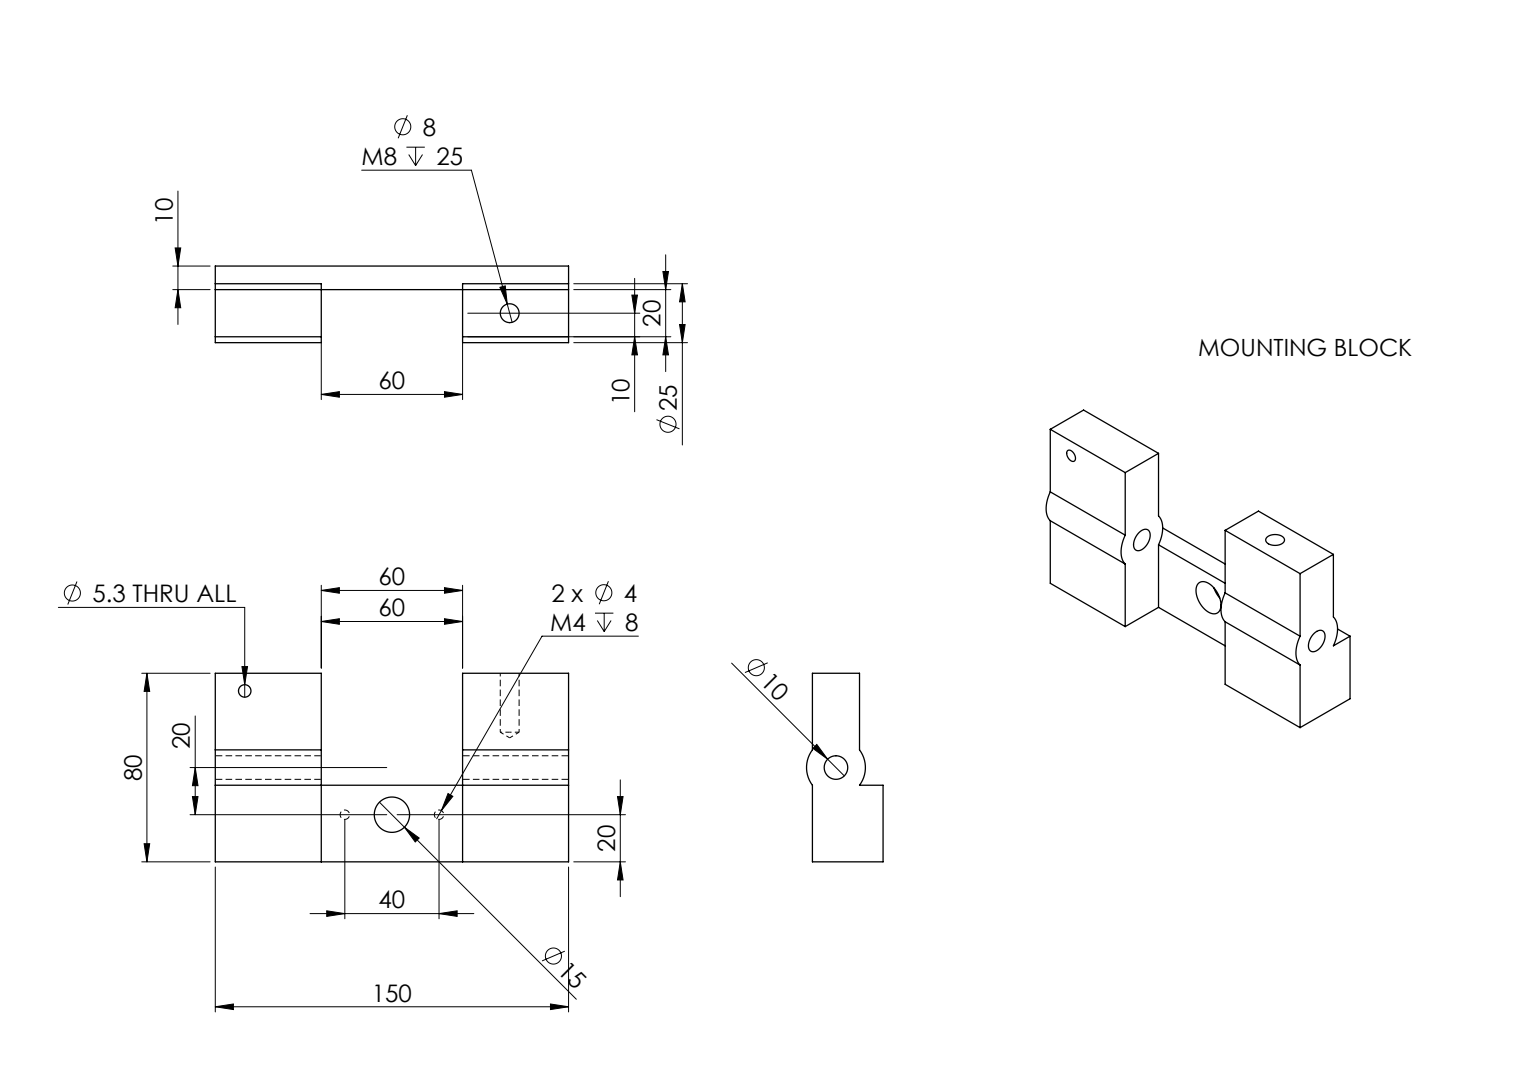
ISO-10303-21;
HEADER;
FILE_DESCRIPTION (('STEP AP214'),
    '1' );
FILE_NAME ('Mounting block.step',
    '2026-10-25T07:12:54',
    ( '' ),
    ( '' ),
    'SwSTEP 2.0',
    'SolidWorks 2026',
    '' );
FILE_SCHEMA (( 'AUTOMOTIVE_DESIGN' ));
ENDSEC;

DATA;
#10=ORIENTED_EDGE ( 'NONE', *, *, #6895, .T. ) ;
#23=DIRECTION ( 'NONE',  ( 1.000000000000000000, 3.469446951953615668E-16, -0.000000000000000000 ) ) ;
#24=DIRECTION ( 'NONE',  ( -1.000000000000000000, 9.251858538542972814E-17, -0.000000000000000000 ) ) ;
#32=FACE_OUTER_BOUND ( 'NONE', #8639, .T. ) ;
#35=VECTOR ( 'NONE', #3248, 1000.000000000000000 ) ;
#47=VECTOR ( 'NONE', #619, 1000.000000000000000 ) ;
#67=EDGE_LOOP ( 'NONE', ( #6510, #1768, #3467, #950 ) ) ;
#82=PLANE ( 'NONE',  #5621 ) ;
#101=ORIENTED_EDGE ( 'NONE', *, *, #5437, .F. ) ;
#111=LINE ( 'NONE', #5314, #1494 ) ;
#116=EDGE_LOOP ( 'NONE', ( #1810, #12426, #10336 ) ) ;
#132=EDGE_CURVE ( 'NONE', #594, #13026, #10926, .T. ) ;
#134=EDGE_CURVE ( 'NONE', #822, #8082, #1591, .T. ) ;
#137=CARTESIAN_POINT ( 'NONE',  ( 50.00000000000000000, 40.00000000000000000, 0.000000000000000000 ) ) ;
#141=CARTESIAN_POINT ( 'NONE',  ( -75.00000000000001421, -5.000000000000025757, 6.123233995736775157E-16 ) ) ;
#152=FACE_OUTER_BOUND ( 'NONE', #7758, .T. ) ;
#163=ADVANCED_FACE ( 'NONE', ( #12857 ), #1236, .F. ) ;
#167=CARTESIAN_POINT ( 'NONE',  ( -75.00000000000001421, -2.602085213965211904E-14, 0.000000000000000000 ) ) ;
#183=FACE_OUTER_BOUND ( 'NONE', #3328, .T. ) ;
#207=VECTOR ( 'NONE', #526, 1000.000000000000000 ) ;
#211=ORIENTED_EDGE ( 'NONE', *, *, #8650, .F. ) ;
#216=EDGE_CURVE ( 'NONE', #11745, #13576, #7487, .T. ) ;
#218=CIRCLE ( 'NONE', #6639, 5.000000000000000000 ) ;
#236=FACE_OUTER_BOUND ( 'NONE', #5614, .T. ) ;
#241=CARTESIAN_POINT ( 'NONE',  ( -30.00000000000000000, 7.499999999999991118, 10.00000000000000000 ) ) ;
#246=VECTOR ( 'NONE', #11169, 1000.000000000000000 ) ;
#251=CARTESIAN_POINT ( 'NONE',  ( 20.00000000000000000, -20.00000000000000000, -12.00000000000000000 ) ) ;
#255=CARTESIAN_POINT ( 'NONE',  ( 75.00000000000001421, 2.602085213965211904E-14, 0.000000000000000000 ) ) ;
#264=ADVANCED_FACE ( 'NONE', ( #3266 ), #5618, .F. ) ;
#293=ORIENTED_EDGE ( 'NONE', *, *, #1456, .F. ) ;
#298=DIRECTION ( 'NONE',  ( 1.000000000000000000, 0.000000000000000000, 0.000000000000000000 ) ) ;
#312=AXIS2_PLACEMENT_3D ( 'NONE', #6238, #11325, #3101 ) ;
#314=DIRECTION ( 'NONE',  ( -0.000000000000000000, -0.000000000000000000, -1.000000000000000000 ) ) ;
#361=ORIENTED_EDGE ( 'NONE', *, *, #4832, .F. ) ;
#366=CARTESIAN_POINT ( 'NONE',  ( -75.00000000000001421, -2.602085213965211904E-14, 0.000000000000000000 ) ) ;
#376=ORIENTED_EDGE ( 'NONE', *, *, #3505, .F. ) ;
#377=ORIENTED_EDGE ( 'NONE', *, *, #754, .F. ) ;
#391=DIRECTION ( 'NONE',  ( 1.000000000000000000, 3.469446951953615175E-16, 0.000000000000000000 ) ) ;
#404=AXIS2_PLACEMENT_3D ( 'NONE', #167, #4383, #2039 ) ;
#419=ORIENTED_EDGE ( 'NONE', *, *, #10834, .F. ) ;
#423=ORIENTED_EDGE ( 'NONE', *, *, #11853, .T. ) ;
#427=EDGE_CURVE ( 'NONE', #5687, #966, #2944, .T. ) ;
#430=AXIS2_PLACEMENT_3D ( 'NONE', #5828, #10990, #3471 ) ;
#440=APPLICATION_CONTEXT ( 'automotive_design' ) ;
#447=CARTESIAN_POINT ( 'NONE',  ( -62.49999999999997158, 32.50000000000001421, 15.00000000000000000 ) ) ;
#448=FACE_OUTER_BOUND ( 'NONE', #5406, .T. ) ;
#450=CARTESIAN_POINT ( 'NONE',  ( 0.000000000000000000, 0.000000000000000000, -10.00000000000000000 ) ) ;
#457=ORIENTED_EDGE ( 'NONE', *, *, #5953, .F. ) ;
#497=EDGE_CURVE ( 'NONE', #9340, #10627, #13638, .T. ) ;
#515=CARTESIAN_POINT ( 'NONE',  ( 30.00000000000000355, -40.00000000000000000, 10.00000000000000000 ) ) ;
#526=DIRECTION ( 'NONE',  ( -0.000000000000000000, -0.000000000000000000, -1.000000000000000000 ) ) ;
#551=FACE_OUTER_BOUND ( 'NONE', #4902, .T. ) ;
#581=CARTESIAN_POINT ( 'NONE',  ( 50.00000000000000000, 40.00000000000000000, 4.000000000000003553 ) ) ;
#583=CARTESIAN_POINT ( 'NONE',  ( -30.00000000000000000, -39.99999999999998579, -10.00000000000000000 ) ) ;
#594=VERTEX_POINT ( 'NONE', #8606 ) ;
#597=CIRCLE ( 'NONE', #11881, 12.50000000000000000 ) ;
#619=DIRECTION ( 'NONE',  ( -0.000000000000000000, -0.000000000000000000, 1.000000000000000000 ) ) ;
#640=DIRECTION ( 'NONE',  ( 1.000000000000000000, 0.000000000000000000, 0.000000000000000000 ) ) ;
#668=EDGE_CURVE ( 'NONE', #3281, #8692, #12777, .T. ) ;
#669=ORIENTED_EDGE ( 'NONE', *, *, #12070, .F. ) ;
#686=VERTEX_POINT ( 'NONE', #2504 ) ;
#699=CARTESIAN_POINT ( 'NONE',  ( 30.00000000000000355, -40.00000000000000000, 0.000000000000000000 ) ) ;
#715=DIRECTION ( 'NONE',  ( -1.000000000000000000, 0.000000000000000000, -0.000000000000000000 ) ) ;
#720=VERTEX_POINT ( 'NONE', #9842 ) ;
#723=ORIENTED_EDGE ( 'NONE', *, *, #9205, .T. ) ;
#726=CIRCLE ( 'NONE', #7603, 2.649999999999985700 ) ;
#738=ORIENTED_EDGE ( 'NONE', *, *, #10743, .T. ) ;
#754=EDGE_CURVE ( 'NONE', #9622, #4847, #5703, .T. ) ;
#771=CARTESIAN_POINT ( 'NONE',  ( 2.449293598294706513E-15, -20.00000000000000000, -20.00000000000000000 ) ) ;
#822=VERTEX_POINT ( 'NONE', #5907 ) ;
#830=AXIS2_PLACEMENT_3D ( 'NONE', #11462, #2962, #13381 ) ;
#859=CARTESIAN_POINT ( 'NONE',  ( 30.00000000000000355, 0.000000000000000000, -10.00000000000000000 ) ) ;
#871=FACE_OUTER_BOUND ( 'NONE', #4942, .T. ) ;
#877=AXIS2_PLACEMENT_3D ( 'NONE', #137, #12911, #3388 ) ;
#885=AXIS2_PLACEMENT_3D ( 'NONE', #1429, #5608, #5539 ) ;
#897=ORIENTED_EDGE ( 'NONE', *, *, #668, .F. ) ;
#931=ADVANCED_FACE ( 'NONE', ( #12055 ), #11004, .F. ) ;
#936=ADVANCED_FACE ( 'NONE', ( #551 ), #3748, .F. ) ;
#939=VECTOR ( 'NONE', #6527, 999.9999999999998863 ) ;
#941=EDGE_LOOP ( 'NONE', ( #8309, #9440 ) ) ;
#944=DIRECTION ( 'NONE',  ( -0.000000000000000000, -0.000000000000000000, -1.000000000000000000 ) ) ;
#950=ORIENTED_EDGE ( 'NONE', *, *, #3505, .T. ) ;
#953=LINE ( 'NONE', #9544, #6686 ) ;
#966=VERTEX_POINT ( 'NONE', #3845 ) ;
#985=ORIENTED_EDGE ( 'NONE', *, *, #7880, .F. ) ;
#991=CARTESIAN_POINT ( 'NONE',  ( -22.00000000000000000, -19.99999999999999289, -20.00000000000000000 ) ) ;
#1004=DIRECTION ( 'NONE',  ( -0.000000000000000000, 1.000000000000000000, -0.000000000000000000 ) ) ;
#1009=VECTOR ( 'NONE', #6135, 1000.000000000000114 ) ;
#1051=DIRECTION ( 'NONE',  ( -1.000000000000000000, 0.000000000000000000, 0.000000000000000000 ) ) ;
#1071=DIRECTION ( 'NONE',  ( 0.000000000000000000, 1.000000000000000000, 0.000000000000000000 ) ) ;
#1091=EDGE_CURVE ( 'NONE', #5946, #5030, #9628, .T. ) ;
#1120=FACE_BOUND ( 'NONE', #6057, .T. ) ;
#1134=FACE_BOUND ( 'NONE', #8492, .T. ) ;
#1135=EDGE_CURVE ( 'NONE', #11879, #2319, #10522, .T. ) ;
#1140=ORIENTED_EDGE ( 'NONE', *, *, #3820, .F. ) ;
#1156=VECTOR ( 'NONE', #12886, 1000.000000000000000 ) ;
#1158=EDGE_CURVE ( 'NONE', #8508, #7078, #7834, .T. ) ;
#1167=LINE ( 'NONE', #8721, #8679 ) ;
#1186=ORIENTED_EDGE ( 'NONE', *, *, #10636, .T. ) ;
#1188=DIRECTION ( 'NONE',  ( -3.469446951953614682E-16, 1.000000000000000000, 0.000000000000000000 ) ) ;
#1196=EDGE_CURVE ( 'NONE', #4847, #8976, #4787, .T. ) ;
#1214=CARTESIAN_POINT ( 'NONE',  ( 0.000000000000000000, 0.000000000000000000, -10.00000000000000000 ) ) ;
#1218=DIRECTION ( 'NONE',  ( 1.000000000000000000, 3.469446951953615175E-16, 0.000000000000000000 ) ) ;
#1226=EDGE_CURVE ( 'NONE', #11270, #10506, #4928, .T. ) ;
#1227=PLANE ( 'NONE',  #1317 ) ;
#1232=ORIENTED_EDGE ( 'NONE', *, *, #1226, .T. ) ;
#1236=CYLINDRICAL_SURFACE ( 'NONE', #7578, 4.000000000000003553 ) ;
#1257=ADVANCED_FACE ( 'NONE', ( #12380 ), #8937, .T. ) ;
#1274=CARTESIAN_POINT ( 'NONE',  ( 30.00000000000000355, -40.00000000000000000, 10.00000000000000000 ) ) ;
#1288=AXIS2_PLACEMENT_3D ( 'NONE', #11344, #5061, #6175 ) ;
#1290=VECTOR ( 'NONE', #1188, 1000.000000000000000 ) ;
#1291=FACE_BOUND ( 'NONE', #2165, .T. ) ;
#1317=AXIS2_PLACEMENT_3D ( 'NONE', #5473, #1427, #6575 ) ;
#1328=EDGE_CURVE ( 'NONE', #11270, #8976, #8325, .T. ) ;
#1340=CARTESIAN_POINT ( 'NONE',  ( 7.500000000000003553, -20.00000000000000000, -10.00000000000000000 ) ) ;
#1349=CARTESIAN_POINT ( 'NONE',  ( -20.00000000000000000, -19.99999999999999289, -12.00000000000000000 ) ) ;
#1375=( NAMED_UNIT ( * ) PLANE_ANGLE_UNIT ( ) SI_UNIT ( $, .RADIAN. ) );
#1382=DIRECTION ( 'NONE',  ( -0.000000000000000000, -0.000000000000000000, 1.000000000000000000 ) ) ;
#1384=VERTEX_POINT ( 'NONE', #10512 ) ;
#1394=AXIS2_PLACEMENT_3D ( 'NONE', #5354, #11635, #6333 ) ;
#1400=ORIENTED_EDGE ( 'NONE', *, *, #11817, .F. ) ;
#1413=CARTESIAN_POINT ( 'NONE',  ( -18.00000000000000355, -19.99999999999999289, -12.00000000000000000 ) ) ;
#1426=EDGE_CURVE ( 'NONE', #11691, #3041, #5274, .T. ) ;
#1427=DIRECTION ( 'NONE',  ( 1.000000000000000000, -0.000000000000000000, 0.000000000000000000 ) ) ;
#1429=CARTESIAN_POINT ( 'NONE',  ( -20.00000000000000000, -19.99999999999999289, -20.00000000000000000 ) ) ;
#1436=EDGE_LOOP ( 'NONE', ( #11212, #8239, #723, #12909 ) ) ;
#1442=DIRECTION ( 'NONE',  ( 0.000000000000000000, -1.000000000000000000, -0.000000000000000000 ) ) ;
#1444=SURFACE_SIDE_STYLE ('',( #12107 ) ) ;
#1452=DIRECTION ( 'NONE',  ( 1.000000000000000000, 3.469446951953615175E-16, 0.000000000000000000 ) ) ;
#1456=EDGE_CURVE ( 'NONE', #11270, #13379, #3187, .T. ) ;
#1461=DIRECTION ( 'NONE',  ( 1.000000000000000000, 3.469446951953615668E-16, -0.000000000000000000 ) ) ;
#1478=FACE_OUTER_BOUND ( 'NONE', #9905, .T. ) ;
#1484=VECTOR ( 'NONE', #9958, 1000.000000000000000 ) ;
#1486=ORIENTED_EDGE ( 'NONE', *, *, #1877, .F. ) ;
#1488=DIRECTION ( 'NONE',  ( 0.8571673013836855759, 1.049727191973305147E-16, -0.5150380737757258576 ) ) ;
#1494=VECTOR ( 'NONE', #3161, 1000.000000000000000 ) ;
#1496=LINE ( 'NONE', #9945, #8636 ) ;
#1523=FACE_OUTER_BOUND ( 'NONE', #4743, .T. ) ;
#1534=MECHANICAL_DESIGN_GEOMETRIC_PRESENTATION_REPRESENTATION('',(#5757),#7318);
#1559=LINE ( 'NONE', #6977, #4152 ) ;
#1591=CIRCLE ( 'NONE', #10443, 2.649999999999985700 ) ;
#1595=ORIENTED_EDGE ( 'NONE', *, *, #6697, .T. ) ;
#1597=DIRECTION ( 'NONE',  ( 1.000000000000000000, -0.000000000000000000, -0.000000000000000000 ) ) ;
#1603=FACE_OUTER_BOUND ( 'NONE', #7658, .T. ) ;
#1624=AXIS2_PLACEMENT_3D ( 'NONE', #5236, #4184, #12612 ) ;
#1631=CARTESIAN_POINT ( 'NONE',  ( 20.00000000000000000, -20.00000000000000000, -20.00000000000000000 ) ) ;
#1633=CARTESIAN_POINT ( 'NONE',  ( -74.99999999999997158, -7.499999999999971578, -20.00000000000000000 ) ) ;
#1634=VECTOR ( 'NONE', #8286, 1000.000000000000000 ) ;
#1637=DIRECTION ( 'NONE',  ( -1.000000000000000000, 0.000000000000000000, 0.000000000000000000 ) ) ;
#1647=ORIENTED_EDGE ( 'NONE', *, *, #668, .T. ) ;
#1649=EDGE_CURVE ( 'NONE', #12919, #5687, #13118, .T. ) ;
#1672=VECTOR ( 'NONE', #7417, 1000.000000000000000 ) ;
#1679=ADVANCED_FACE ( 'NONE', ( #871 ), #8157, .F. ) ;
#1701=CARTESIAN_POINT ( 'NONE',  ( 75.00000000000002842, -39.99999999999998579, -10.00000000000000000 ) ) ;
#1702=EDGE_CURVE ( 'NONE', #13026, #10076, #2059, .T. ) ;
#1703=ORIENTED_EDGE ( 'NONE', *, *, #10554, .T. ) ;
#1707=CARTESIAN_POINT ( 'NONE',  ( -75.00000000000001421, 4.999999999999974243, 0.000000000000000000 ) ) ;
#1712=FACE_OUTER_BOUND ( 'NONE', #12953, .T. ) ;
#1714=ORIENTED_EDGE ( 'NONE', *, *, #9304, .F. ) ;
#1747=CARTESIAN_POINT ( 'NONE',  ( 50.00000000000000000, 15.00000000000000000, 0.000000000000000000 ) ) ;
#1754=VERTEX_POINT ( 'NONE', #1274 ) ;
#1768=ORIENTED_EDGE ( 'NONE', *, *, #9656, .F. ) ;
#1778=CARTESIAN_POINT ( 'NONE',  ( 20.00000000000000000, -20.00000000000000000, -20.00000000000000000 ) ) ;
#1788=ORIENTED_EDGE ( 'NONE', *, *, #132, .T. ) ;
#1801=CIRCLE ( 'NONE', #3579, 7.500000000000000888 ) ;
#1810=ORIENTED_EDGE ( 'NONE', *, *, #10510, .F. ) ;
#1818=CARTESIAN_POINT ( 'NONE',  ( 75.00000000000001421, -7.499999999999975131, 10.00000000000000000 ) ) ;
#1839=ADVANCED_FACE ( 'NONE', ( #9600 ), #10702, .F. ) ;
#1845=ORIENTED_EDGE ( 'NONE', *, *, #11259, .F. ) ;
#1846=AXIS2_PLACEMENT_3D ( 'NONE', #11714, #8479, #7506 ) ;
#1861=ORIENTED_EDGE ( 'NONE', *, *, #216, .F. ) ;
#1877=EDGE_CURVE ( 'NONE', #13576, #11319, #3241, .T. ) ;
#1915=VERTEX_POINT ( 'NONE', #2324 ) ;
#1918=DIRECTION ( 'NONE',  ( -1.000000000000000000, 0.000000000000000000, 0.000000000000000000 ) ) ;
#1924=CARTESIAN_POINT ( 'NONE',  ( -74.99999999999997158, 40.00000000000001421, 10.00000000000000000 ) ) ;
#1942=ORIENTED_EDGE ( 'NONE', *, *, #3391, .T. ) ;
#1944=UNCERTAINTY_MEASURE_WITH_UNIT (LENGTH_MEASURE( 1.000000000000000082E-05 ), #6590, 'distance_accuracy_value', 'NONE');
#1945=ORIENTED_EDGE ( 'NONE', *, *, #9317, .T. ) ;
#1949=EDGE_CURVE ( 'NONE', #3416, #8098, #11368, .T. ) ;
#1952=EDGE_CURVE ( 'NONE', #3196, #4232, #3412, .T. ) ;
#1958=CIRCLE ( 'NONE', #12979, 5.000000000000000000 ) ;
#1993=PLANE ( 'NONE',  #11909 ) ;
#1995=DIRECTION ( 'NONE',  ( 1.000000000000000000, 3.469446951953615175E-16, 0.000000000000000000 ) ) ;
#2039=DIRECTION ( 'NONE',  ( 0.000000000000000000, 1.000000000000000000, 0.000000000000000000 ) ) ;
#2040=LINE ( 'NONE', #991, #13547 ) ;
#2041=ADVANCED_FACE ( 'NONE', ( #5797, #448 ), #4685, .F. ) ;
#2049=AXIS2_PLACEMENT_3D ( 'NONE', #4295, #11820, #3393 ) ;
#2050=ORIENTED_EDGE ( 'NONE', *, *, #13637, .T. ) ;
#2059=LINE ( 'NONE', #9190, #7185 ) ;
#2084=CIRCLE ( 'NONE', #4091, 5.000000000000000000 ) ;
#2093=CARTESIAN_POINT ( 'NONE',  ( -75.00000000000001421, 4.999999999999974243, 0.000000000000000000 ) ) ;
#2094=LINE ( 'NONE', #8465, #1009 ) ;
#2102=VERTEX_POINT ( 'NONE', #1413 ) ;
#2104=DIRECTION ( 'NONE',  ( 0.000000000000000000, 0.000000000000000000, -1.000000000000000000 ) ) ;
#2110=LINE ( 'NONE', #6358, #6956 ) ;
#2115=VECTOR ( 'NONE', #8203, 1000.000000000000000 ) ;
#2117=DIRECTION ( 'NONE',  ( 0.000000000000000000, 0.000000000000000000, 1.000000000000000000 ) ) ;
#2119=CARTESIAN_POINT ( 'NONE',  ( 0.000000000000000000, 0.000000000000000000, 10.00000000000000000 ) ) ;
#2152=DIRECTION ( 'NONE',  ( -0.000000000000000000, -0.000000000000000000, -1.000000000000000000 ) ) ;
#2164=DIRECTION ( 'NONE',  ( 0.000000000000000000, 1.000000000000000000, 0.000000000000000000 ) ) ;
#2165=EDGE_LOOP ( 'NONE', ( #7409, #4103 ) ) ;
#2173=DIRECTION ( 'NONE',  ( -0.000000000000000000, -0.000000000000000000, -1.000000000000000000 ) ) ;
#2179=CIRCLE ( 'NONE', #3511, 12.50000000000000000 ) ;
#2249=VERTEX_POINT ( 'NONE', #10812 ) ;
#2253=DIRECTION ( 'NONE',  ( -0.000000000000000000, -1.000000000000000000, -0.000000000000000000 ) ) ;
#2288=CYLINDRICAL_SURFACE ( 'NONE', #11511, 4.000000000000003553 ) ;
#2304=CARTESIAN_POINT ( 'NONE',  ( -74.99999999999998579, -2.602085213965210642E-14, 0.000000000000000000 ) ) ;
#2316=CARTESIAN_POINT ( 'NONE',  ( -74.99999999999997158, -39.99999999999998579, 10.00000000000000000 ) ) ;
#2318=PRODUCT_DEFINITION_CONTEXT ( 'detailed design', #440, 'design' ) ;
#2319=VERTEX_POINT ( 'NONE', #241 ) ;
#2324=CARTESIAN_POINT ( 'NONE',  ( -22.00000000000000000, -19.99999999999999289, -20.00000000000000000 ) ) ;
#2328=DIRECTION ( 'NONE',  ( 0.000000000000000000, 0.000000000000000000, -1.000000000000000000 ) ) ;
#2335=VECTOR ( 'NONE', #2798, 1000.000000000000000 ) ;
#2353=CARTESIAN_POINT ( 'NONE',  ( -74.99999999999997158, -7.499999999999971578, -20.00000000000000000 ) ) ;
#2366=ORIENTED_EDGE ( 'NONE', *, *, #10588, .F. ) ;
#2370=CARTESIAN_POINT ( 'NONE',  ( -30.00000000000000000, -7.500000000000005329, -10.00000000000000711 ) ) ;
#2404=CARTESIAN_POINT ( 'NONE',  ( -75.00000000000001421, -2.602085213965211904E-14, 0.000000000000000000 ) ) ;
#2415=ORIENTED_EDGE ( 'NONE', *, *, #1328, .F. ) ;
#2416=ORIENTED_EDGE ( 'NONE', *, *, #3382, .T. ) ;
#2421=PRESENTATION_STYLE_ASSIGNMENT (( #3402 ) ) ;
#2461=DIRECTION ( 'NONE',  ( -0.000000000000000000, -0.000000000000000000, -1.000000000000000000 ) ) ;
#2471=DIRECTION ( 'NONE',  ( 0.8571673013836855759, 1.049727191973305147E-16, -0.5150380737757258576 ) ) ;
#2474=CARTESIAN_POINT ( 'NONE',  ( 18.00000000000000355, -20.00000000000000000, -20.00000000000000000 ) ) ;
#2483=CARTESIAN_POINT ( 'NONE',  ( 50.00000000000000000, 15.00000000000000000, 4.000000000000003553 ) ) ;
#2494=( LENGTH_UNIT ( ) NAMED_UNIT ( * ) SI_UNIT ( .MILLI., .METRE. ) );
#2504=CARTESIAN_POINT ( 'NONE',  ( -29.99999999999999645, 40.00000000000000000, 10.00000000000000000 ) ) ;
#2509=CYLINDRICAL_SURFACE ( 'NONE', #12395, 5.000000000000000000 ) ;
#2527=LINE ( 'NONE', #10962, #246 ) ;
#2536=EDGE_CURVE ( 'NONE', #12922, #5946, #12064, .T. ) ;
#2595=DIRECTION ( 'NONE',  ( 1.000000000000000000, 3.469446951953615175E-16, 0.000000000000000000 ) ) ;
#2607=ORIENTED_EDGE ( 'NONE', *, *, #6781, .F. ) ;
#2610=DIRECTION ( 'NONE',  ( 1.000000000000000000, 0.000000000000000000, 0.000000000000000000 ) ) ;
#2644=AXIS2_PLACEMENT_3D ( 'NONE', #6226, #2173, #8420 ) ;
#2664=LINE ( 'NONE', #12142, #9310 ) ;
#2665=EDGE_CURVE ( 'NONE', #4232, #7288, #5165, .T. ) ;
#2714=EDGE_CURVE ( 'NONE', #9523, #10506, #3071, .T. ) ;
#2716=EDGE_CURVE ( 'NONE', #5028, #3281, #2094, .T. ) ;
#2738=EDGE_CURVE ( 'NONE', #2102, #11896, #9569, .T. ) ;
#2739=CARTESIAN_POINT ( 'NONE',  ( -74.99999999999998579, -2.602085213965210642E-14, 0.000000000000000000 ) ) ;
#2743=PLANE ( 'NONE',  #3538 ) ;
#2767=ORIENTED_EDGE ( 'NONE', *, *, #8814, .T. ) ;
#2781=LINE ( 'NONE', #4792, #6884 ) ;
#2796=VECTOR ( 'NONE', #10173, 1000.000000000000000 ) ;
#2798=DIRECTION ( 'NONE',  ( -0.000000000000000000, 1.000000000000000000, -0.000000000000000000 ) ) ;
#2831=DIRECTION ( 'NONE',  ( 0.000000000000000000, 0.000000000000000000, 1.000000000000000000 ) ) ;
#2869=AXIS2_PLACEMENT_3D ( 'NONE', #5399, #1995, #12704 ) ;
#2887=ORIENTED_EDGE ( 'NONE', *, *, #1196, .T. ) ;
#2897=AXIS2_PLACEMENT_3D ( 'NONE', #1214, #10631, #6366 ) ;
#2899=EDGE_CURVE ( 'NONE', #3196, #5220, #6596, .T. ) ;
#2905=EDGE_LOOP ( 'NONE', ( #5183, #1140, #4287, #10711, #12022, #9220, #8658, #6657, #6582 ) ) ;
#2919=AXIS2_PLACEMENT_3D ( 'NONE', #771, #5022, #9228 ) ;
#2944=LINE ( 'NONE', #7168, #4339 ) ;
#2945=ORIENTED_EDGE ( 'NONE', *, *, #754, .T. ) ;
#2946=ORIENTED_EDGE ( 'NONE', *, *, #12963, .T. ) ;
#2948=FACE_OUTER_BOUND ( 'NONE', #13091, .T. ) ;
#2959=ORIENTED_EDGE ( 'NONE', *, *, #12763, .T. ) ;
#2962=DIRECTION ( 'NONE',  ( 0.000000000000000000, 0.000000000000000000, -1.000000000000000000 ) ) ;
#3039=EDGE_CURVE ( 'NONE', #10021, #3041, #6864, .T. ) ;
#3041=VERTEX_POINT ( 'NONE', #8943 ) ;
#3056=ORIENTED_EDGE ( 'NONE', *, *, #9519, .F. ) ;
#3060=ORIENTED_EDGE ( 'NONE', *, *, #11753, .T. ) ;
#3069=ADVANCED_FACE ( 'NONE', ( #3750 ), #11067, .F. ) ;
#3071=LINE ( 'NONE', #6277, #12931 ) ;
#3076=ADVANCED_FACE ( 'NONE', ( #1523 ), #9900, .T. ) ;
#3101=DIRECTION ( 'NONE',  ( 0.000000000000000000, 1.776356839400250267E-15, 1.000000000000000000 ) ) ;
#3108=COLOUR_RGB ( '',0.8941176470588234615, 0.8941176470588234615, 0.8941176470588234615 ) ;
#3126=ORIENTED_EDGE ( 'NONE', *, *, #3820, .T. ) ;
#3136=DIRECTION ( 'NONE',  ( 0.000000000000000000, 0.000000000000000000, 1.000000000000000000 ) ) ;
#3152=CARTESIAN_POINT ( 'NONE',  ( 20.00000000000000000, -20.00000000000000000, -12.00000000000000000 ) ) ;
#3161=DIRECTION ( 'NONE',  ( 0.000000000000000000, 1.000000000000000000, 0.000000000000000000 ) ) ;
#3169=CARTESIAN_POINT ( 'NONE',  ( 0.000000000000000000, 0.000000000000000000, -20.00000000000000000 ) ) ;
#3182=ORIENTED_EDGE ( 'NONE', *, *, #10900, .F. ) ;
#3186=CARTESIAN_POINT ( 'NONE',  ( 75.00000000000001421, -39.99999999999998579, -20.00000000000000000 ) ) ;
#3187=LINE ( 'NONE', #6383, #1672 ) ;
#3195=AXIS2_PLACEMENT_3D ( 'NONE', #12897, #9801, #1071 ) ;
#3196=VERTEX_POINT ( 'NONE', #5003 ) ;
#3199=AXIS2_PLACEMENT_3D ( 'NONE', #11749, #7538, #10647 ) ;
#3204=LINE ( 'NONE', #4370, #8653 ) ;
#3238=LINE ( 'NONE', #11864, #7262 ) ;
#3240=FACE_OUTER_BOUND ( 'NONE', #5268, .T. ) ;
#3241=LINE ( 'NONE', #12762, #9605 ) ;
#3244=CARTESIAN_POINT ( 'NONE',  ( 75.00000000000000000, 40.00000000000000000, 10.00000000000000000 ) ) ;
#3248=DIRECTION ( 'NONE',  ( -0.000000000000000000, -1.000000000000000000, -0.000000000000000000 ) ) ;
#3266=FACE_OUTER_BOUND ( 'NONE', #4135, .T. ) ;
#3267=( LENGTH_UNIT ( ) NAMED_UNIT ( * ) SI_UNIT ( .MILLI., .METRE. ) );
#3268=LINE ( 'NONE', #5426, #3537 ) ;
#3275=CARTESIAN_POINT ( 'NONE',  ( -18.00000000000000355, -19.99999999999999289, -20.00000000000000000 ) ) ;
#3281=VERTEX_POINT ( 'NONE', #8580 ) ;
#3285=CARTESIAN_POINT ( 'NONE',  ( -62.49999999999997158, 32.50000000000001421, -10.00000000000000178 ) ) ;
#3313=PRODUCT_DEFINITION_FORMATION_WITH_SPECIFIED_SOURCE ( 'ANY', '', #12721, .NOT_KNOWN. ) ;
#3328=EDGE_LOOP ( 'NONE', ( #6851, #7021, #2945, #2887 ) ) ;
#3337=DIRECTION ( 'NONE',  ( -1.000000000000000000, 0.000000000000000000, -0.000000000000000000 ) ) ;
#3344=EDGE_CURVE ( 'NONE', #11691, #12157, #10654, .T. ) ;
#3351=AXIS2_PLACEMENT_3D ( 'NONE', #7533, #10568, #4283 ) ;
#3382=EDGE_CURVE ( 'NONE', #11879, #2249, #1167, .T. ) ;
#3388=DIRECTION ( 'NONE',  ( 0.000000000000000000, 0.000000000000000000, 1.000000000000000000 ) ) ;
#3391=EDGE_CURVE ( 'NONE', #9340, #13026, #8015, .T. ) ;
#3393=DIRECTION ( 'NONE',  ( 0.000000000000000000, 0.000000000000000000, 1.000000000000000000 ) ) ;
#3401=CARTESIAN_POINT ( 'NONE',  ( 75.00000000000001421, -7.499999999999971578, -20.00000000000000000 ) ) ;
#3402=SURFACE_STYLE_USAGE ( .BOTH. , #1444 ) ;
#3403=VECTOR ( 'NONE', #1597, 1000.000000000000000 ) ;
#3412=CIRCLE ( 'NONE', #9382, 7.500000000000000888 ) ;
#3416=VERTEX_POINT ( 'NONE', #141 ) ;
#3419=EDGE_LOOP ( 'NONE', ( #7619, #8388, #6978, #10492 ) ) ;
#3421=CARTESIAN_POINT ( 'NONE',  ( 50.00000000000000000, 15.00000000000000000, -4.000000000000003553 ) ) ;
#3447=LINE ( 'NONE', #5330, #35 ) ;
#3456=AXIS2_PLACEMENT_3D ( 'NONE', #10931, #3337, #6530 ) ;
#3459=EDGE_CURVE ( 'NONE', #594, #9340, #3800, .T. ) ;
#3467=ORIENTED_EDGE ( 'NONE', *, *, #12766, .T. ) ;
#3471=DIRECTION ( 'NONE',  ( 1.000000000000000000, 0.000000000000000000, 0.000000000000000000 ) ) ;
#3505=EDGE_CURVE ( 'NONE', #1915, #11896, #8250, .T. ) ;
#3507=FACE_OUTER_BOUND ( 'NONE', #5479, .T. ) ;
#3511=AXIS2_PLACEMENT_3D ( 'NONE', #2304, #11648, #7315 ) ;
#3514=AXIS2_PLACEMENT_3D ( 'NONE', #1747, #7986, #8198 ) ;
#3520=DIRECTION ( 'NONE',  ( -0.000000000000000000, -0.000000000000000000, -1.000000000000000000 ) ) ;
#3534=ORIENTED_EDGE ( 'NONE', *, *, #9097, .F. ) ;
#3537=VECTOR ( 'NONE', #4369, 1000.000000000000000 ) ;
#3538=AXIS2_PLACEMENT_3D ( 'NONE', #11242, #12349, #715 ) ;
#3539=CARTESIAN_POINT ( 'NONE',  ( -75.00000000000001421, 4.999999999999974243, 0.000000000000000000 ) ) ;
#3546=DIRECTION ( 'NONE',  ( -1.000000000000000000, -3.469446951953615175E-16, -0.000000000000000000 ) ) ;
#3566=DIRECTION ( 'NONE',  ( -9.251858538542972814E-17, -1.000000000000000000, 0.000000000000000000 ) ) ;
#3568=ORIENTED_EDGE ( 'NONE', *, *, #10310, .T. ) ;
#3569=ORIENTED_EDGE ( 'NONE', *, *, #9506, .F. ) ;
#3579=AXIS2_PLACEMENT_3D ( 'NONE', #9347, #11486, #8766 ) ;
#3581=PLANE ( 'NONE',  #9925 ) ;
#3608=CLOSED_SHELL ( 'NONE', ( #936, #11073, #4298, #10590, #931, #13593, #163, #11669, #11377, #1839, #2041, #11261, #12385, #12706, #7019, #13489, #7630, #3076, #8981, #3630, #7094, #12062, #264, #10905, #12878, #9841, #1257, #9735, #3832, #10141, #8726, #3069, #11882, #9071, #6213, #7037, #1679, #6700, #9353, #5072 ) ) ;
#3609=VECTOR ( 'NONE', #11901, 1000.000000000000000 ) ;
#3618=DIRECTION ( 'NONE',  ( 0.000000000000000000, 1.000000000000000000, 0.000000000000000000 ) ) ;
#3630=ADVANCED_FACE ( 'NONE', ( #1134, #1712 ), #12434, .F. ) ;
#3637=VERTEX_POINT ( 'NONE', #5958 ) ;
#3641=DIRECTION ( 'NONE',  ( 0.000000000000000000, 1.776356839400250465E-15, 1.000000000000000000 ) ) ;
#3674=ORIENTED_EDGE ( 'NONE', *, *, #9986, .T. ) ;
#3675=DIRECTION ( 'NONE',  ( 1.000000000000000000, -0.000000000000000000, -0.000000000000000000 ) ) ;
#3677=CARTESIAN_POINT ( 'NONE',  ( -74.99999999999998579, -2.602085213965210642E-14, 0.000000000000000000 ) ) ;
#3684=EDGE_LOOP ( 'NONE', ( #361, #6347, #3568, #9134, #2607, #8117, #13363, #6671 ) ) ;
#3699=ORIENTED_EDGE ( 'NONE', *, *, #9643, .T. ) ;
#3703=AXIS2_PLACEMENT_3D ( 'NONE', #7294, #10526, #9558 ) ;
#3707=DIRECTION ( 'NONE',  ( -0.000000000000000000, 0.000000000000000000, -1.000000000000000000 ) ) ;
#3715=ORIENTED_EDGE ( 'NONE', *, *, #7033, .T. ) ;
#3748=CONICAL_SURFACE ( 'NONE', #9494, 1.999999999999998224, 1.029744259999999745 ) ;
#3750=FACE_OUTER_BOUND ( 'NONE', #4865, .T. ) ;
#3756=LINE ( 'NONE', #13147, #12459 ) ;
#3797=LINE ( 'NONE', #1707, #4408 ) ;
#3800=LINE ( 'NONE', #2483, #4259 ) ;
#3807=VERTEX_POINT ( 'NONE', #9917 ) ;
#3814=DIRECTION ( 'NONE',  ( 1.000000000000000000, -0.000000000000000000, -0.000000000000000000 ) ) ;
#3820=EDGE_CURVE ( 'NONE', #2249, #7376, #11793, .T. ) ;
#3832=ADVANCED_FACE ( 'NONE', ( #13023 ), #8691, .F. ) ;
#3838=VERTEX_POINT ( 'NONE', #10693 ) ;
#3845=CARTESIAN_POINT ( 'NONE',  ( -29.99999999999999645, 40.00000000000000000, -9.999999999999998224 ) ) ;
#3867=CARTESIAN_POINT ( 'NONE',  ( -30.00000000000000000, 7.499999999999996447, -9.999999999999994671 ) ) ;
#3877=DIRECTION ( 'NONE',  ( -0.000000000000000000, -0.000000000000000000, 1.000000000000000000 ) ) ;
#3899=DIRECTION ( 'NONE',  ( -0.000000000000000000, -0.000000000000000000, 1.000000000000000000 ) ) ;
#3942=FACE_OUTER_BOUND ( 'NONE', #9610, .T. ) ;
#3945=DIRECTION ( 'NONE',  ( 1.000000000000000000, 3.469446951953615668E-16, -0.000000000000000000 ) ) ;
#3960=CARTESIAN_POINT ( 'NONE',  ( -75.00000000000001421, -5.000000000000025757, 6.123233995736766282E-16 ) ) ;
#3967=ORIENTED_EDGE ( 'NONE', *, *, #12275, .F. ) ;
#3993=EDGE_LOOP ( 'NONE', ( #12436, #12510, #4380, #6170 ) ) ;
#4006=CARTESIAN_POINT ( 'NONE',  ( -20.00000000000000000, -19.99999999999999289, -20.00000000000000000 ) ) ;
#4031=ORIENTED_EDGE ( 'NONE', *, *, #2716, .T. ) ;
#4035=( NAMED_UNIT ( * ) SI_UNIT ( $, .STERADIAN. ) SOLID_ANGLE_UNIT ( ) );
#4054=LINE ( 'NONE', #8279, #4070 ) ;
#4070=VECTOR ( 'NONE', #9174, 1000.000000000000000 ) ;
#4091=AXIS2_PLACEMENT_3D ( 'NONE', #8441, #7413, #11619 ) ;
#4103=ORIENTED_EDGE ( 'NONE', *, *, #10500, .F. ) ;
#4135=EDGE_LOOP ( 'NONE', ( #11354, #12004, #6285, #5584, #12786, #6442 ) ) ;
#4138=ORIENTED_EDGE ( 'NONE', *, *, #3391, .F. ) ;
#4149=VERTEX_POINT ( 'NONE', #8063 ) ;
#4152=VECTOR ( 'NONE', #2471, 1000.000000000000114 ) ;
#4171=LINE ( 'NONE', #8394, #10471 ) ;
#4184=DIRECTION ( 'NONE',  ( -0.000000000000000000, -0.000000000000000000, -1.000000000000000000 ) ) ;
#4195=CIRCLE ( 'NONE', #10398, 5.000000000000000000 ) ;
#4199=CARTESIAN_POINT ( 'NONE',  ( -74.99999999999997158, -7.499999999999971578, -20.00000000000000000 ) ) ;
#4221=CARTESIAN_POINT ( 'NONE',  ( -74.99999999999997158, -39.99999999999998579, -20.00000000000000000 ) ) ;
#4230=AXIS2_PLACEMENT_3D ( 'NONE', #447, #12691, #10760 ) ;
#4232=VERTEX_POINT ( 'NONE', #8271 ) ;
#4256=ORIENTED_EDGE ( 'NONE', *, *, #9890, .T. ) ;
#4259=VECTOR ( 'NONE', #4774, 999.9999999999998863 ) ;
#4281=DIRECTION ( 'NONE',  ( -1.000000000000000000, 9.251858538542972814E-17, -0.000000000000000000 ) ) ;
#4283=DIRECTION ( 'NONE',  ( 0.000000000000000000, 0.000000000000000000, 1.000000000000000000 ) ) ;
#4287=ORIENTED_EDGE ( 'NONE', *, *, #11603, .F. ) ;
#4295=CARTESIAN_POINT ( 'NONE',  ( 50.00000000000000000, 15.00000000000000000, 0.000000000000000000 ) ) ;
#4298=ADVANCED_FACE ( 'NONE', ( #13635 ), #13550, .F. ) ;
#4304=CIRCLE ( 'NONE', #11809, 5.000000000000000000 ) ;
#4306=FACE_OUTER_BOUND ( 'NONE', #7074, .T. ) ;
#4332=CARTESIAN_POINT ( 'NONE',  ( -62.49999999999997158, 32.50000000000001421, 10.00000000000000000 ) ) ;
#4339=VECTOR ( 'NONE', #2164, 1000.000000000000000 ) ;
#4341=ORIENTED_EDGE ( 'NONE', *, *, #5151, .T. ) ;
#4369=DIRECTION ( 'NONE',  ( -0.000000000000000000, -0.000000000000000000, 1.000000000000000000 ) ) ;
#4370=CARTESIAN_POINT ( 'NONE',  ( -22.00000000000000000, -19.99999999999999289, -12.00000000000000000 ) ) ;
#4376=CARTESIAN_POINT ( 'NONE',  ( 75.00000000000001421, -7.499999999999971578, -20.00000000000000000 ) ) ;
#4380=ORIENTED_EDGE ( 'NONE', *, *, #10500, .T. ) ;
#4383=DIRECTION ( 'NONE',  ( 1.000000000000000000, 3.469446951953615668E-16, -0.000000000000000000 ) ) ;
#4397=EDGE_LOOP ( 'NONE', ( #12005, #3534 ) ) ;
#4407=CARTESIAN_POINT ( 'NONE',  ( 75.00000000000001421, 7.500000000000027534, -10.00000000000000000 ) ) ;
#4408=VECTOR ( 'NONE', #12163, 1000.000000000000000 ) ;
#4448=ORIENTED_EDGE ( 'NONE', *, *, #1649, .T. ) ;
#4480=DIRECTION ( 'NONE',  ( 0.000000000000000000, 1.000000000000000000, 0.000000000000000000 ) ) ;
#4507=CONICAL_SURFACE ( 'NONE', #1394, 4.000000000000003553, 1.029744260000001077 ) ;
#4556=ORIENTED_EDGE ( 'NONE', *, *, #9097, .T. ) ;
#4574=DIRECTION ( 'NONE',  ( -1.000000000000000000, 0.000000000000000000, 0.000000000000000000 ) ) ;
#4607=EDGE_LOOP ( 'NONE', ( #10427, #7252, #9828, #293 ) ) ;
#4619=AXIS2_PLACEMENT_3D ( 'NONE', #5305, #13640, #6541 ) ;
#4631=FACE_OUTER_BOUND ( 'NONE', #2905, .T. ) ;
#4640=EDGE_CURVE ( 'NONE', #8508, #5565, #8005, .T. ) ;
#4648=LINE ( 'NONE', #2353, #7962 ) ;
#4660=EDGE_CURVE ( 'NONE', #7376, #3807, #10485, .T. ) ;
#4683=DIRECTION ( 'NONE',  ( 1.000000000000000000, 3.469446951953615175E-16, 0.000000000000000000 ) ) ;
#4685=PLANE ( 'NONE',  #7346 ) ;
#4689=CIRCLE ( 'NONE', #2919, 7.500000000000000888 ) ;
#4701=VECTOR ( 'NONE', #3546, 1000.000000000000000 ) ;
#4704=DIRECTION ( 'NONE',  ( -0.000000000000000000, -0.000000000000000000, 1.000000000000000000 ) ) ;
#4727=PRODUCT_DEFINITION ( 'UNKNOWN', '', #3313, #2318 ) ;
#4731=ORIENTED_EDGE ( 'NONE', *, *, #12070, .T. ) ;
#4743=EDGE_LOOP ( 'NONE', ( #6316, #9826, #7860, #3569 ) ) ;
#4748=CIRCLE ( 'NONE', #5202, 1.999999999999998224 ) ;
#4754=EDGE_CURVE ( 'NONE', #5030, #10987, #2110, .T. ) ;
#4774=DIRECTION ( 'NONE',  ( 0.000000000000000000, 0.5150380737757248584, 0.8571673013836862420 ) ) ;
#4782=AXIS2_PLACEMENT_3D ( 'NONE', #3677, #6998, #13401 ) ;
#4787=LINE ( 'NONE', #7066, #2796 ) ;
#4792=CARTESIAN_POINT ( 'NONE',  ( 75.00000000000001421, -7.499999999999971578, -10.00000000000000000 ) ) ;
#4825=VECTOR ( 'NONE', #314, 1000.000000000000000 ) ;
#4832=EDGE_CURVE ( 'NONE', #11691, #1754, #10328, .T. ) ;
#4847=VERTEX_POINT ( 'NONE', #1818 ) ;
#4851=LINE ( 'NONE', #8012, #10339 ) ;
#4865=EDGE_LOOP ( 'NONE', ( #8241, #5100, #4341, #11197 ) ) ;
#4867=CIRCLE ( 'NONE', #2869, 12.50000000000000000 ) ;
#4902=EDGE_LOOP ( 'NONE', ( #985, #4920, #3674 ) ) ;
#4920=ORIENTED_EDGE ( 'NONE', *, *, #10510, .T. ) ;
#4921=ORIENTED_EDGE ( 'NONE', *, *, #1952, .F. ) ;
#4928=LINE ( 'NONE', #8106, #8547 ) ;
#4932=AXIS2_PLACEMENT_3D ( 'NONE', #9077, #1452, #3618 ) ;
#4942=EDGE_LOOP ( 'NONE', ( #5457, #897, #2767, #12205 ) ) ;
#4965=VECTOR ( 'NONE', #11573, 1000.000000000000000 ) ;
#4976=ORIENTED_EDGE ( 'NONE', *, *, #1649, .F. ) ;
#4992=ORIENTED_EDGE ( 'NONE', *, *, #9519, .T. ) ;
#5003=CARTESIAN_POINT ( 'NONE',  ( -7.499999999999998224, -20.00000000000000000, -20.00000000000000000 ) ) ;
#5012=ORIENTED_EDGE ( 'NONE', *, *, #8650, .T. ) ;
#5013=EDGE_CURVE ( 'NONE', #4232, #3196, #4689, .T. ) ;
#5022=DIRECTION ( 'NONE',  ( 0.000000000000000000, 0.000000000000000000, 1.000000000000000000 ) ) ;
#5028=VERTEX_POINT ( 'NONE', #6339 ) ;
#5029=ORIENTED_EDGE ( 'NONE', *, *, #13527, .T. ) ;
#5030=VERTEX_POINT ( 'NONE', #4376 ) ;
#5053=VECTOR ( 'NONE', #3877, 1000.000000000000000 ) ;
#5058=ORIENTED_EDGE ( 'NONE', *, *, #1456, .T. ) ;
#5061=DIRECTION ( 'NONE',  ( 0.000000000000000000, 0.000000000000000000, 1.000000000000000000 ) ) ;
#5072=ADVANCED_FACE ( 'NONE', ( #5364 ), #6466, .F. ) ;
#5077=ORIENTED_EDGE ( 'NONE', *, *, #7819, .F. ) ;
#5086=SHAPE_DEFINITION_REPRESENTATION ( #10744, #10956 ) ;
#5095=CIRCLE ( 'NONE', #2644, 1.999999999999998224 ) ;
#5100=ORIENTED_EDGE ( 'NONE', *, *, #11853, .F. ) ;
#5132=ORIENTED_EDGE ( 'NONE', *, *, #3382, .F. ) ;
#5150=ORIENTED_EDGE ( 'NONE', *, *, #427, .T. ) ;
#5151=EDGE_CURVE ( 'NONE', #8098, #10200, #9497, .T. ) ;
#5165=LINE ( 'NONE', #7160, #5456 ) ;
#5183=ORIENTED_EDGE ( 'NONE', *, *, #6781, .T. ) ;
#5190=DIRECTION ( 'NONE',  ( -0.000000000000000000, -0.000000000000000000, -1.000000000000000000 ) ) ;
#5202=AXIS2_PLACEMENT_3D ( 'NONE', #11396, #5190, #1918 ) ;
#5210=DIRECTION ( 'NONE',  ( -1.000000000000000000, 9.251858538542972814E-17, -0.000000000000000000 ) ) ;
#5220=VERTEX_POINT ( 'NONE', #8873 ) ;
#5236=CARTESIAN_POINT ( 'NONE',  ( 20.00000000000000000, -20.00000000000000000, -12.00000000000000000 ) ) ;
#5237=ORIENTED_EDGE ( 'NONE', *, *, #10900, .T. ) ;
#5254=ORIENTED_EDGE ( 'NONE', *, *, #11259, .T. ) ;
#5268=EDGE_LOOP ( 'NONE', ( #5405, #12646, #419, #2366 ) ) ;
#5272=CARTESIAN_POINT ( 'NONE',  ( 75.00000000000002842, -39.99999999999998579, 10.00000000000000000 ) ) ;
#5274=LINE ( 'NONE', #12516, #13602 ) ;
#5305=CARTESIAN_POINT ( 'NONE',  ( 75.00000000000002842, -39.99999999999998579, 10.00000000000000000 ) ) ;
#5314=CARTESIAN_POINT ( 'NONE',  ( -29.99999999999999645, 0.000000000000000000, -10.00000000000000000 ) ) ;
#5327=LINE ( 'NONE', #9336, #9716 ) ;
#5330=CARTESIAN_POINT ( 'NONE',  ( -29.99999999999999645, -40.00000000000000000, 10.00000000000000000 ) ) ;
#5336=DIRECTION ( 'NONE',  ( 1.000000000000000000, 3.469446951953615175E-16, 0.000000000000000000 ) ) ;
#5339=DIRECTION ( 'NONE',  ( -1.000000000000000000, 0.000000000000000000, 0.000000000000000000 ) ) ;
#5344=DIRECTION ( 'NONE',  ( -1.000000000000000000, 0.000000000000000000, 0.000000000000000000 ) ) ;
#5354=CARTESIAN_POINT ( 'NONE',  ( 50.00000000000000000, 15.00000000000000000, 0.000000000000000000 ) ) ;
#5364=FACE_OUTER_BOUND ( 'NONE', #116, .T. ) ;
#5383=DIRECTION ( 'NONE',  ( -1.000000000000000000, 0.000000000000000000, 0.000000000000000000 ) ) ;
#5392=DIRECTION ( 'NONE',  ( -1.000000000000000000, 0.000000000000000000, 0.000000000000000000 ) ) ;
#5399=CARTESIAN_POINT ( 'NONE',  ( 75.00000000000001421, 2.602085213965211904E-14, 0.000000000000000000 ) ) ;
#5405=ORIENTED_EDGE ( 'NONE', *, *, #1158, .F. ) ;
#5406=EDGE_LOOP ( 'NONE', ( #457, #11971, #12458, #101 ) ) ;
#5426=CARTESIAN_POINT ( 'NONE',  ( -29.99999999999999645, 40.00000000000000000, 0.000000000000000000 ) ) ;
#5433=DIRECTION ( 'NONE',  ( -1.000000000000000000, 0.000000000000000000, 0.000000000000000000 ) ) ;
#5437=EDGE_CURVE ( 'NONE', #12919, #3041, #2781, .T. ) ;
#5456=VECTOR ( 'NONE', #12540, 1000.000000000000000 ) ;
#5457=ORIENTED_EDGE ( 'NONE', *, *, #10999, .F. ) ;
#5459=FACE_BOUND ( 'NONE', #9985, .T. ) ;
#5473=CARTESIAN_POINT ( 'NONE',  ( -30.00000000000000000, -40.00000000000000000, 12.50000000000000000 ) ) ;
#5479=EDGE_LOOP ( 'NONE', ( #6283, #4031, #1647 ) ) ;
#5520=PLANE ( 'NONE',  #2897 ) ;
#5539=DIRECTION ( 'NONE',  ( -1.000000000000000000, 0.000000000000000000, 0.000000000000000000 ) ) ;
#5542=CARTESIAN_POINT ( 'NONE',  ( 75.00000000000001421, -39.99999999999998579, -10.00000000000000000 ) ) ;
#5560=EDGE_CURVE ( 'NONE', #13026, #9340, #8440, .T. ) ;
#5565=VERTEX_POINT ( 'NONE', #6568 ) ;
#5583=ORIENTED_EDGE ( 'NONE', *, *, #10588, .T. ) ;
#5584=ORIENTED_EDGE ( 'NONE', *, *, #7033, .F. ) ;
#5597=VECTOR ( 'NONE', #6725, 1000.000000000000000 ) ;
#5608=DIRECTION ( 'NONE',  ( -0.000000000000000000, -0.000000000000000000, -1.000000000000000000 ) ) ;
#5614=EDGE_LOOP ( 'NONE', ( #9870, #4992, #7760, #4731 ) ) ;
#5615=ORIENTED_EDGE ( 'NONE', *, *, #2714, .T. ) ;
#5617=EDGE_CURVE ( 'NONE', #686, #2319, #3447, .T. ) ;
#5618=PLANE ( 'NONE',  #6275 ) ;
#5621=AXIS2_PLACEMENT_3D ( 'NONE', #10527, #9560, #9626 ) ;
#5660=CARTESIAN_POINT ( 'NONE',  ( 2.449293598294706513E-15, -20.00000000000000000, -20.00000000000000000 ) ) ;
#5669=ORIENTED_EDGE ( 'NONE', *, *, #4640, .F. ) ;
#5673=APPLICATION_CONTEXT ( 'automotive_design' ) ;
#5687=VERTEX_POINT ( 'NONE', #3867 ) ;
#5689=CARTESIAN_POINT ( 'NONE',  ( 50.00000000000000000, 40.00000000000000000, 0.000000000000000000 ) ) ;
#5692=CARTESIAN_POINT ( 'NONE',  ( -74.99999999999998579, 7.499999999999975131, -10.00000000000000000 ) ) ;
#5696=ADVANCED_BREP_SHAPE_REPRESENTATION ( '', ( #10159, #430 ), #11706 ) ;
#5699=EDGE_CURVE ( 'NONE', #10200, #7846, #1958, .T. ) ;
#5703=LINE ( 'NONE', #8806, #1290 ) ;
#5718=EDGE_LOOP ( 'NONE', ( #8915, #4138, #9379, #5012 ) ) ;
#5730=AXIS2_PLACEMENT_3D ( 'NONE', #3152, #10543, #1051 ) ;
#5731=FACE_OUTER_BOUND ( 'NONE', #12870, .T. ) ;
#5741=EDGE_CURVE ( 'NONE', #8082, #822, #7275, .T. ) ;
#5757=STYLED_ITEM ( 'NONE', ( #2421 ), #5696 ) ;
#5758=CARTESIAN_POINT ( 'NONE',  ( 75.00000000000002842, -39.99999999999998579, 10.00000000000000000 ) ) ;
#5771=EDGE_LOOP ( 'NONE', ( #7058, #9758 ) ) ;
#5772=DIRECTION ( 'NONE',  ( -0.000000000000000000, -0.000000000000000000, 1.000000000000000000 ) ) ;
#5797=FACE_BOUND ( 'NONE', #5771, .T. ) ;
#5822=VERTEX_POINT ( 'NONE', #6004 ) ;
#5825=ORIENTED_EDGE ( 'NONE', *, *, #427, .F. ) ;
#5828=CARTESIAN_POINT ( 'NONE',  ( 0.000000000000000000, 0.000000000000000000, 0.000000000000000000 ) ) ;
#5838=DIRECTION ( 'NONE',  ( 1.000000000000000000, 0.000000000000000000, 0.000000000000000000 ) ) ;
#5863=LINE ( 'NONE', #13226, #4825 ) ;
#5896=LINE ( 'NONE', #8244, #12405 ) ;
#5903=CARTESIAN_POINT ( 'NONE',  ( -75.00000000000001421, -2.602085213965211904E-14, 0.000000000000000000 ) ) ;
#5907=CARTESIAN_POINT ( 'NONE',  ( -59.84999999999998721, 32.50000000000001421, 10.00000000000000000 ) ) ;
#5930=CYLINDRICAL_SURFACE ( 'NONE', #4230, 2.649999999999985700 ) ;
#5946=VERTEX_POINT ( 'NONE', #4199 ) ;
#5949=LINE ( 'NONE', #9123, #207 ) ;
#5953=EDGE_CURVE ( 'NONE', #12157, #12919, #111, .T. ) ;
#5958=CARTESIAN_POINT ( 'NONE',  ( -22.00000000000000000, -19.99999999999999289, -12.00000000000000000 ) ) ;
#5964=ORIENTED_EDGE ( 'NONE', *, *, #2716, .F. ) ;
#6001=DIRECTION ( 'NONE',  ( -1.000000000000000000, 0.000000000000000000, -0.000000000000000000 ) ) ;
#6004=CARTESIAN_POINT ( 'NONE',  ( 75.00000000000001421, 5.000000000000025757, 0.000000000000000000 ) ) ;
#6027=FACE_OUTER_BOUND ( 'NONE', #67, .T. ) ;
#6057=EDGE_LOOP ( 'NONE', ( #8168, #1400 ) ) ;
#6101=CARTESIAN_POINT ( 'NONE',  ( 75.00000000000000000, 40.00000000000000000, -10.00000000000000000 ) ) ;
#6106=ORIENTED_EDGE ( 'NONE', *, *, #5013, .F. ) ;
#6109=CARTESIAN_POINT ( 'NONE',  ( 30.00000000000000355, -39.99999999999998579, -10.00000000000000178 ) ) ;
#6129=PRODUCT_CONTEXT ( 'NONE', #5673, 'mechanical' ) ;
#6135=DIRECTION ( 'NONE',  ( -0.8571673013836855759, 0.000000000000000000, -0.5150380737757258576 ) ) ;
#6170=ORIENTED_EDGE ( 'NONE', *, *, #5151, .F. ) ;
#6175=DIRECTION ( 'NONE',  ( 1.000000000000000000, 0.000000000000000000, 0.000000000000000000 ) ) ;
#6180=LINE ( 'NONE', #3186, #9944 ) ;
#6213=ADVANCED_FACE ( 'NONE', ( #1603 ), #10576, .F. ) ;
#6226=CARTESIAN_POINT ( 'NONE',  ( -20.00000000000000000, -19.99999999999999289, -12.00000000000000000 ) ) ;
#6230=VERTEX_POINT ( 'NONE', #11157 ) ;
#6238=CARTESIAN_POINT ( 'NONE',  ( -30.00000000000000000, -1.040834085586084257E-14, 0.000000000000000000 ) ) ;
#6246=VERTEX_POINT ( 'NONE', #11087 ) ;
#6254=DIRECTION ( 'NONE',  ( -1.000000000000000000, 0.000000000000000000, 0.000000000000000000 ) ) ;
#6260=CONICAL_SURFACE ( 'NONE', #10862, 1.999999999999998224, 1.029744259999999745 ) ;
#6275=AXIS2_PLACEMENT_3D ( 'NONE', #3401, #1442, #6588 ) ;
#6277=CARTESIAN_POINT ( 'NONE',  ( -74.99999999999997158, 40.00000000000001421, 10.00000000000000000 ) ) ;
#6283=ORIENTED_EDGE ( 'NONE', *, *, #10554, .F. ) ;
#6285=ORIENTED_EDGE ( 'NONE', *, *, #3039, .F. ) ;
#6286=ORIENTED_EDGE ( 'NONE', *, *, #4754, .F. ) ;
#6304=CARTESIAN_POINT ( 'NONE',  ( 30.00000000000000000, -7.499999999999991118, 10.00000000000000000 ) ) ;
#6316=ORIENTED_EDGE ( 'NONE', *, *, #3039, .T. ) ;
#6317=CYLINDRICAL_SURFACE ( 'NONE', #12987, 7.500000000000000888 ) ;
#6319=LINE ( 'NONE', #4221, #7354 ) ;
#6333=DIRECTION ( 'NONE',  ( 0.000000000000000000, 0.000000000000000000, 1.000000000000000000 ) ) ;
#6339=CARTESIAN_POINT ( 'NONE',  ( 20.00000000000000000, -20.00000000000000000, -10.79827876554711530 ) ) ;
#6347=ORIENTED_EDGE ( 'NONE', *, *, #3344, .T. ) ;
#6358=CARTESIAN_POINT ( 'NONE',  ( 75.00000000000001421, -7.499999999999971578, -20.00000000000000000 ) ) ;
#6366=DIRECTION ( 'NONE',  ( -1.000000000000000000, 0.000000000000000000, -0.000000000000000000 ) ) ;
#6383=CARTESIAN_POINT ( 'NONE',  ( -74.99999999999998579, 7.499999999999975131, 10.00000000000000000 ) ) ;
#6442=ORIENTED_EDGE ( 'NONE', *, *, #8224, .T. ) ;
#6443=DIRECTION ( 'NONE',  ( 0.000000000000000000, 1.000000000000000000, 0.000000000000000000 ) ) ;
#6459=EDGE_LOOP ( 'NONE', ( #10228, #8013, #1861, #3056 ) ) ;
#6466=CONICAL_SURFACE ( 'NONE', #6899, 1.999999999999998224, 1.029744259999999745 ) ;
#6469=DIRECTION ( 'NONE',  ( -0.000000000000000000, -0.000000000000000000, -1.000000000000000000 ) ) ;
#6480=AXIS2_PLACEMENT_3D ( 'NONE', #5903, #7969, #11140 ) ;
#6495=UNCERTAINTY_MEASURE_WITH_UNIT (LENGTH_MEASURE( 1.000000000000000082E-05 ), #3267, 'distance_accuracy_value', 'NONE');
#6510=ORIENTED_EDGE ( 'NONE', *, *, #2738, .F. ) ;
#6512=CYLINDRICAL_SURFACE ( 'NONE', #3199, 7.500000000000000888 ) ;
#6527=DIRECTION ( 'NONE',  ( 1.049727191973306010E-16, 0.5150380737757248584, -0.8571673013836862420 ) ) ;
#6530=DIRECTION ( 'NONE',  ( 0.000000000000000000, 1.776356839400250465E-15, -1.000000000000000000 ) ) ;
#6532=DIRECTION ( 'NONE',  ( -0.000000000000000000, 1.000000000000000000, -0.000000000000000000 ) ) ;
#6541=DIRECTION ( 'NONE',  ( 3.469446951953615175E-16, -1.000000000000000000, 0.000000000000000000 ) ) ;
#6568=CARTESIAN_POINT ( 'NONE',  ( 30.00000000000000355, 40.00000000000000000, -9.999999999999998224 ) ) ;
#6575=DIRECTION ( 'NONE',  ( 0.000000000000000000, 0.000000000000000000, -1.000000000000000000 ) ) ;
#6582=ORIENTED_EDGE ( 'NONE', *, *, #2536, .F. ) ;
#6588=DIRECTION ( 'NONE',  ( 0.000000000000000000, 0.000000000000000000, -1.000000000000000000 ) ) ;
#6590=( LENGTH_UNIT ( ) NAMED_UNIT ( * ) SI_UNIT ( .MILLI., .METRE. ) );
#6596=LINE ( 'NONE', #8599, #7366 ) ;
#6621=EDGE_CURVE ( 'NONE', #6230, #13042, #5896, .T. ) ;
#6622=UNCERTAINTY_MEASURE_WITH_UNIT (LENGTH_MEASURE( 1.000000000000000082E-05 ), #2494, 'distance_accuracy_value', 'NONE');
#6625=DIRECTION ( 'NONE',  ( -1.000000000000000000, 0.000000000000000000, -0.000000000000000000 ) ) ;
#6639=AXIS2_PLACEMENT_3D ( 'NONE', #255, #1218, #4480 ) ;
#6657=ORIENTED_EDGE ( 'NONE', *, *, #8224, .F. ) ;
#6663=DIRECTION ( 'NONE',  ( -1.000000000000000000, 0.000000000000000000, -0.000000000000000000 ) ) ;
#6670=DIRECTION ( 'NONE',  ( -0.000000000000000000, -0.000000000000000000, -1.000000000000000000 ) ) ;
#6671=ORIENTED_EDGE ( 'NONE', *, *, #13165, .F. ) ;
#6676=EDGE_CURVE ( 'NONE', #13379, #9523, #13611, .T. ) ;
#6686=VECTOR ( 'NONE', #5210, 1000.000000000000000 ) ;
#6691=ORIENTED_EDGE ( 'NONE', *, *, #5013, .T. ) ;
#6692=DIRECTION ( 'NONE',  ( -0.000000000000000000, -0.000000000000000000, -1.000000000000000000 ) ) ;
#6697=EDGE_CURVE ( 'NONE', #7288, #5220, #1801, .T. ) ;
#6700=ADVANCED_FACE ( 'NONE', ( #3507 ), #6260, .F. ) ;
#6713=EDGE_CURVE ( 'NONE', #966, #13576, #953, .T. ) ;
#6724=ORIENTED_EDGE ( 'NONE', *, *, #5560, .F. ) ;
#6725=DIRECTION ( 'NONE',  ( -0.000000000000000000, -0.000000000000000000, -1.000000000000000000 ) ) ;
#6742=DIRECTION ( 'NONE',  ( 0.000000000000000000, 1.000000000000000000, 0.000000000000000000 ) ) ;
#6781=EDGE_CURVE ( 'NONE', #12922, #7376, #6319, .T. ) ;
#6795=CARTESIAN_POINT ( 'NONE',  ( 30.00000000000000000, 1.040834085586084888E-14, 0.000000000000000000 ) ) ;
#6807=CIRCLE ( 'NONE', #12104, 5.000000000000000000 ) ;
#6817=EDGE_LOOP ( 'NONE', ( #12338, #10351, #10371, #9100 ) ) ;
#6832=ORIENTED_EDGE ( 'NONE', *, *, #3459, .T. ) ;
#6843=CIRCLE ( 'NONE', #7742, 1.999999999999998224 ) ;
#6851=ORIENTED_EDGE ( 'NONE', *, *, #9890, .F. ) ;
#6854=CIRCLE ( 'NONE', #877, 4.000000000000003553 ) ;
#6864=LINE ( 'NONE', #9003, #4701 ) ;
#6866=CIRCLE ( 'NONE', #885, 1.999999999999998224 ) ;
#6884=VECTOR ( 'NONE', #12575, 1000.000000000000000 ) ;
#6892=DIRECTION ( 'NONE',  ( -0.000000000000000000, -1.000000000000000000, -0.000000000000000000 ) ) ;
#6893=LINE ( 'NONE', #7800, #7129 ) ;
#6895=EDGE_CURVE ( 'NONE', #11319, #5687, #6893, .T. ) ;
#6899=AXIS2_PLACEMENT_3D ( 'NONE', #7497, #6469, #5433 ) ;
#6908=PLANE ( 'NONE',  #9163 ) ;
#6920=ORIENTED_EDGE ( 'NONE', *, *, #497, .F. ) ;
#6955=ORIENTED_EDGE ( 'NONE', *, *, #6621, .F. ) ;
#6956=VECTOR ( 'NONE', #12559, 1000.000000000000000 ) ;
#6977=CARTESIAN_POINT ( 'NONE',  ( 22.00000000000000000, -20.00000000000000000, -12.00000000000000000 ) ) ;
#6978=ORIENTED_EDGE ( 'NONE', *, *, #11817, .T. ) ;
#6998=DIRECTION ( 'NONE',  ( 1.000000000000000000, 3.469446951953615175E-16, 0.000000000000000000 ) ) ;
#7019=ADVANCED_FACE ( 'NONE', ( #12210 ), #8835, .T. ) ;
#7021=ORIENTED_EDGE ( 'NONE', *, *, #13165, .T. ) ;
#7033=EDGE_CURVE ( 'NONE', #5030, #10021, #2527, .T. ) ;
#7037=ADVANCED_FACE ( 'NONE', ( #1478 ), #5930, .F. ) ;
#7038=AXIS2_PLACEMENT_3D ( 'NONE', #12006, #6692, #12206 ) ;
#7058=ORIENTED_EDGE ( 'NONE', *, *, #6697, .F. ) ;
#7066=CARTESIAN_POINT ( 'NONE',  ( -74.99999999999998579, -7.500000000000027534, 10.00000000000000000 ) ) ;
#7074=EDGE_LOOP ( 'NONE', ( #4976, #7151, #7958, #10 ) ) ;
#7078=VERTEX_POINT ( 'NONE', #4407 ) ;
#7094=ADVANCED_FACE ( 'NONE', ( #3240 ), #5520, .T. ) ;
#7129=VECTOR ( 'NONE', #4683, 1000.000000000000000 ) ;
#7130=EDGE_LOOP ( 'NONE', ( #12824, #11288 ) ) ;
#7133=ORIENTED_EDGE ( 'NONE', *, *, #1135, .F. ) ;
#7134=CARTESIAN_POINT ( 'NONE',  ( -74.99999999999997158, 40.00000000000001421, 10.00000000000000000 ) ) ;
#7151=ORIENTED_EDGE ( 'NONE', *, *, #13093, .F. ) ;
#7160=CARTESIAN_POINT ( 'NONE',  ( 7.500000000000003553, -20.00000000000000000, -20.00000000000000000 ) ) ;
#7168=CARTESIAN_POINT ( 'NONE',  ( -29.99999999999999645, 0.000000000000000000, -10.00000000000000000 ) ) ;
#7185=VECTOR ( 'NONE', #8227, 1000.000000000000000 ) ;
#7238=ORIENTED_EDGE ( 'NONE', *, *, #3459, .F. ) ;
#7251=EDGE_CURVE ( 'NONE', #11745, #6246, #2664, .T. ) ;
#7252=ORIENTED_EDGE ( 'NONE', *, *, #1196, .F. ) ;
#7257=ORIENTED_EDGE ( 'NONE', *, *, #13527, .F. ) ;
#7262=VECTOR ( 'NONE', #12757, 1000.000000000000000 ) ;
#7275=CIRCLE ( 'NONE', #11671, 2.649999999999985700 ) ;
#7283=CIRCLE ( 'NONE', #1288, 7.500000000000000888 ) ;
#7288=VERTEX_POINT ( 'NONE', #1340 ) ;
#7294=CARTESIAN_POINT ( 'NONE',  ( -74.99999999999998579, -2.602085213965210642E-14, 0.000000000000000000 ) ) ;
#7315=DIRECTION ( 'NONE',  ( 0.000000000000000000, 1.000000000000000000, 0.000000000000000000 ) ) ;
#7318=( GEOMETRIC_REPRESENTATION_CONTEXT ( 3 ) GLOBAL_UNCERTAINTY_ASSIGNED_CONTEXT ( ( #1944 ) ) GLOBAL_UNIT_ASSIGNED_CONTEXT ( ( #6590, #1375, #13065 ) ) REPRESENTATION_CONTEXT ( 'NONE', 'WORKASPACE' ) );
#7346=AXIS2_PLACEMENT_3D ( 'NONE', #8906, #3707, #13100 ) ;
#7348=DIRECTION ( 'NONE',  ( -0.000000000000000000, -0.000000000000000000, 1.000000000000000000 ) ) ;
#7354=VECTOR ( 'NONE', #7348, 1000.000000000000000 ) ;
#7364=CARTESIAN_POINT ( 'NONE',  ( -29.99999999999999645, -40.00000000000000000, 10.00000000000000000 ) ) ;
#7366=VECTOR ( 'NONE', #1382, 1000.000000000000000 ) ;
#7376=VERTEX_POINT ( 'NONE', #11449 ) ;
#7379=CARTESIAN_POINT ( 'NONE',  ( -74.99999999999997158, 7.499999999999971578, -10.00000000000000000 ) ) ;
#7409=ORIENTED_EDGE ( 'NONE', *, *, #5699, .F. ) ;
#7413=DIRECTION ( 'NONE',  ( 1.000000000000000000, 3.469446951953615175E-16, 0.000000000000000000 ) ) ;
#7417=DIRECTION ( 'NONE',  ( 1.000000000000000000, 3.469446951953615175E-16, 0.000000000000000000 ) ) ;
#7428=CARTESIAN_POINT ( 'NONE',  ( -74.99999999999997158, 40.00000000000001421, -10.00000000000000000 ) ) ;
#7457=PLANE ( 'NONE',  #10773 ) ;
#7487=LINE ( 'NONE', #11692, #5597 ) ;
#7497=CARTESIAN_POINT ( 'NONE',  ( -20.00000000000000000, -19.99999999999999289, -12.00000000000000000 ) ) ;
#7506=DIRECTION ( 'NONE',  ( -1.000000000000000000, 0.000000000000000000, -0.000000000000000000 ) ) ;
#7516=DIRECTION ( 'NONE',  ( 0.000000000000000000, 0.000000000000000000, -1.000000000000000000 ) ) ;
#7533=CARTESIAN_POINT ( 'NONE',  ( 50.00000000000000000, 15.00000000000000000, 0.000000000000000000 ) ) ;
#7538=DIRECTION ( 'NONE',  ( -0.000000000000000000, -0.000000000000000000, 1.000000000000000000 ) ) ;
#7549=EDGE_LOOP ( 'NONE', ( #5964, #1703, #5254 ) ) ;
#7553=ORIENTED_EDGE ( 'NONE', *, *, #5741, .F. ) ;
#7569=ORIENTED_EDGE ( 'NONE', *, *, #1949, .T. ) ;
#7578=AXIS2_PLACEMENT_3D ( 'NONE', #5689, #11765, #9761 ) ;
#7603=AXIS2_PLACEMENT_3D ( 'NONE', #3285, #2104, #9578 ) ;
#7609=AXIS2_PLACEMENT_3D ( 'NONE', #8967, #7930, #7801 ) ;
#7610=CARTESIAN_POINT ( 'NONE',  ( 22.00000000000000000, -20.00000000000000000, -12.00000000000000000 ) ) ;
#7618=ORIENTED_EDGE ( 'NONE', *, *, #4832, .T. ) ;
#7619=ORIENTED_EDGE ( 'NONE', *, *, #12159, .T. ) ;
#7623=CARTESIAN_POINT ( 'NONE',  ( -62.49999999999997158, 32.50000000000001421, 10.00000000000000000 ) ) ;
#7624=LINE ( 'NONE', #11828, #5053 ) ;
#7630=ADVANCED_FACE ( 'NONE', ( #9846 ), #2509, .F. ) ;
#7635=DIRECTION ( 'NONE',  ( -0.000000000000000000, -0.000000000000000000, -1.000000000000000000 ) ) ;
#7658=EDGE_LOOP ( 'NONE', ( #10287, #6832, #1942 ) ) ;
#7659=FACE_OUTER_BOUND ( 'NONE', #6817, .T. ) ;
#7742=AXIS2_PLACEMENT_3D ( 'NONE', #1349, #2461, #8702 ) ;
#7745=DIRECTION ( 'NONE',  ( -3.469446951953614682E-16, 1.000000000000000000, 0.000000000000000000 ) ) ;
#7758=EDGE_LOOP ( 'NONE', ( #7238, #1788, #8223 ) ) ;
#7760=ORIENTED_EDGE ( 'NONE', *, *, #7251, .T. ) ;
#7794=VECTOR ( 'NONE', #5344, 1000.000000000000000 ) ;
#7797=CYLINDRICAL_SURFACE ( 'NONE', #7038, 1.999999999999998224 ) ;
#7800=CARTESIAN_POINT ( 'NONE',  ( -74.99999999999998579, 7.499999999999975131, -10.00000000000000000 ) ) ;
#7801=DIRECTION ( 'NONE',  ( 0.000000000000000000, 1.000000000000000000, 0.000000000000000000 ) ) ;
#7819=EDGE_CURVE ( 'NONE', #4149, #822, #9011, .T. ) ;
#7822=AXIS2_PLACEMENT_3D ( 'NONE', #11448, #10410, #6001 ) ;
#7831=( NAMED_UNIT ( * ) SI_UNIT ( $, .STERADIAN. ) SOLID_ANGLE_UNIT ( ) );
#7834=LINE ( 'NONE', #5692, #9860 ) ;
#7844=ORIENTED_EDGE ( 'NONE', *, *, #10834, .T. ) ;
#7846=VERTEX_POINT ( 'NONE', #9156 ) ;
#7860=ORIENTED_EDGE ( 'NONE', *, *, #1158, .T. ) ;
#7880=EDGE_CURVE ( 'NONE', #11165, #3637, #3204, .T. ) ;
#7890=DIRECTION ( 'NONE',  ( -1.000000000000000000, 0.000000000000000000, 0.000000000000000000 ) ) ;
#7897=DIRECTION ( 'NONE',  ( 0.000000000000000000, 0.000000000000000000, 1.000000000000000000 ) ) ;
#7898=FILL_AREA_STYLE ('',( #11829 ) ) ;
#7930=DIRECTION ( 'NONE',  ( 1.000000000000000000, 3.469446951953615175E-16, 0.000000000000000000 ) ) ;
#7941=EDGE_LOOP ( 'NONE', ( #7133, #5029, #9639, #9343, #4448, #5150, #2050, #8933 ) ) ;
#7946=FACE_BOUND ( 'NONE', #9409, .T. ) ;
#7958=ORIENTED_EDGE ( 'NONE', *, *, #11285, .T. ) ;
#7962=VECTOR ( 'NONE', #13066, 1000.000000000000000 ) ;
#7969=DIRECTION ( 'NONE',  ( 1.000000000000000000, 3.469446951953615668E-16, -0.000000000000000000 ) ) ;
#7978=LINE ( 'NONE', #13012, #3403 ) ;
#7979=CARTESIAN_POINT ( 'NONE',  ( -59.84999999999998721, 32.50000000000001421, 15.00000000000000000 ) ) ;
#7986=DIRECTION ( 'NONE',  ( -0.000000000000000000, 1.000000000000000000, -0.000000000000000000 ) ) ;
#7996=FACE_OUTER_BOUND ( 'NONE', #1436, .T. ) ;
#8005=LINE ( 'NONE', #859, #1634 ) ;
#8012=CARTESIAN_POINT ( 'NONE',  ( -18.00000000000000355, -19.99999999999999289, -12.00000000000000000 ) ) ;
#8013=ORIENTED_EDGE ( 'NONE', *, *, #6713, .T. ) ;
#8015=CIRCLE ( 'NONE', #2049, 4.000000000000003553 ) ;
#8059=CARTESIAN_POINT ( 'NONE',  ( -74.99999999999997158, -7.499999999999971578, -20.00000000000000000 ) ) ;
#8063=CARTESIAN_POINT ( 'NONE',  ( -59.84999999999998721, 32.50000000000001421, -10.00000000000000178 ) ) ;
#8068=AXIS2_PLACEMENT_3D ( 'NONE', #2119, #11865, #6625 ) ;
#8082=VERTEX_POINT ( 'NONE', #12925 ) ;
#8094=CARTESIAN_POINT ( 'NONE',  ( -30.00000000000000000, -1.040834085586084257E-14, 0.000000000000000000 ) ) ;
#8098=VERTEX_POINT ( 'NONE', #3539 ) ;
#8106=CARTESIAN_POINT ( 'NONE',  ( 30.00000000000000355, -40.00000000000000000, 10.00000000000000000 ) ) ;
#8117=ORIENTED_EDGE ( 'NONE', *, *, #8566, .F. ) ;
#8136=MECHANICAL_DESIGN_GEOMETRIC_PRESENTATION_REPRESENTATION('',(#13629),#11434);
#8147=EDGE_LOOP ( 'NONE', ( #12303, #6106, #11057, #1595 ) ) ;
#8157=CYLINDRICAL_SURFACE ( 'NONE', #10258, 1.999999999999998224 ) ;
#8168=ORIENTED_EDGE ( 'NONE', *, *, #9643, .F. ) ;
#8188=ORIENTED_EDGE ( 'NONE', *, *, #10999, .T. ) ;
#8198=DIRECTION ( 'NONE',  ( 0.000000000000000000, 0.000000000000000000, 1.000000000000000000 ) ) ;
#8203=DIRECTION ( 'NONE',  ( -0.000000000000000000, 1.000000000000000000, -0.000000000000000000 ) ) ;
#8204=EDGE_LOOP ( 'NONE', ( #9236, #3967 ) ) ;
#8223=ORIENTED_EDGE ( 'NONE', *, *, #5560, .T. ) ;
#8224=EDGE_CURVE ( 'NONE', #5946, #10489, #4648, .T. ) ;
#8226=VECTOR ( 'NONE', #12960, 1000.000000000000000 ) ;
#8227=DIRECTION ( 'NONE',  ( -0.000000000000000000, 1.000000000000000000, -0.000000000000000000 ) ) ;
#8229=DIRECTION ( 'NONE',  ( -0.000000000000000000, -0.000000000000000000, -1.000000000000000000 ) ) ;
#8239=ORIENTED_EDGE ( 'NONE', *, *, #2738, .T. ) ;
#8241=ORIENTED_EDGE ( 'NONE', *, *, #13451, .F. ) ;
#8244=CARTESIAN_POINT ( 'NONE',  ( -75.00000000000001421, -5.000000000000025757, 6.123233995736766282E-16 ) ) ;
#8250=CIRCLE ( 'NONE', #10667, 1.999999999999998224 ) ;
#8271=CARTESIAN_POINT ( 'NONE',  ( 7.500000000000003553, -20.00000000000000000, -20.00000000000000000 ) ) ;
#8279=CARTESIAN_POINT ( 'NONE',  ( 75.00000000000000000, 40.00000000000000000, 10.00000000000000000 ) ) ;
#8286=DIRECTION ( 'NONE',  ( 0.000000000000000000, 1.000000000000000000, 0.000000000000000000 ) ) ;
#8309=ORIENTED_EDGE ( 'NONE', *, *, #134, .T. ) ;
#8325=CIRCLE ( 'NONE', #11839, 12.50000000000000000 ) ;
#8354=DIRECTION ( 'NONE',  ( 1.000000000000000000, 0.000000000000000000, 0.000000000000000000 ) ) ;
#8375=DIRECTION ( 'NONE',  ( 1.000000000000000000, 3.469446951953615175E-16, 0.000000000000000000 ) ) ;
#8388=ORIENTED_EDGE ( 'NONE', *, *, #6621, .T. ) ;
#8394=CARTESIAN_POINT ( 'NONE',  ( 30.00000000000000355, 40.00000000000000000, 0.000000000000000000 ) ) ;
#8407=VECTOR ( 'NONE', #8969, 1000.000000000000000 ) ;
#8414=CARTESIAN_POINT ( 'NONE',  ( -74.99999999999997158, -39.99999999999998579, -20.00000000000000000 ) ) ;
#8420=DIRECTION ( 'NONE',  ( -1.000000000000000000, 0.000000000000000000, 0.000000000000000000 ) ) ;
#8432=DIRECTION ( 'NONE',  ( 0.000000000000000000, 1.000000000000000000, 0.000000000000000000 ) ) ;
#8440=CIRCLE ( 'NONE', #3351, 4.000000000000003553 ) ;
#8441=CARTESIAN_POINT ( 'NONE',  ( 75.00000000000001421, 2.602085213965211904E-14, 0.000000000000000000 ) ) ;
#8458=FACE_BOUND ( 'NONE', #4397, .T. ) ;
#8465=CARTESIAN_POINT ( 'NONE',  ( 18.00000000000000355, -20.00000000000000000, -12.00000000000000000 ) ) ;
#8479=DIRECTION ( 'NONE',  ( 0.000000000000000000, 0.000000000000000000, -1.000000000000000000 ) ) ;
#8492=EDGE_LOOP ( 'NONE', ( #211, #3182 ) ) ;
#8506=AXIS2_PLACEMENT_3D ( 'NONE', #2404, #5336, #6443 ) ;
#8508=VERTEX_POINT ( 'NONE', #11681 ) ;
#8528=DIRECTION ( 'NONE',  ( -1.000000000000000000, 0.000000000000000000, 0.000000000000000000 ) ) ;
#8547=VECTOR ( 'NONE', #11277, 1000.000000000000000 ) ;
#8566=EDGE_CURVE ( 'NONE', #10987, #12922, #6180, .T. ) ;
#8580=CARTESIAN_POINT ( 'NONE',  ( 18.00000000000000355, -20.00000000000000000, -12.00000000000000000 ) ) ;
#8592=DIRECTION ( 'NONE',  ( 1.000000000000000000, 3.469446951953615175E-16, 0.000000000000000000 ) ) ;
#8599=CARTESIAN_POINT ( 'NONE',  ( -7.499999999999998224, -20.00000000000000000, -20.00000000000000000 ) ) ;
#8605=AXIS2_PLACEMENT_3D ( 'NONE', #12430, #8229, #10498 ) ;
#8606=CARTESIAN_POINT ( 'NONE',  ( 50.00000000000000000, 12.59655753109423237, 0.000000000000000000 ) ) ;
#8622=DIRECTION ( 'NONE',  ( 1.000000000000000000, -9.251858538542972814E-17, 0.000000000000000000 ) ) ;
#8625=ORIENTED_EDGE ( 'NONE', *, *, #11002, .F. ) ;
#8632=CARTESIAN_POINT ( 'NONE',  ( 75.00000000000002842, -39.99999999999998579, 10.00000000000000000 ) ) ;
#8636=VECTOR ( 'NONE', #4704, 1000.000000000000000 ) ;
#8639=EDGE_LOOP ( 'NONE', ( #12841, #1186, #377, #11539, #6286, #3715, #11675, #5583, #11283 ) ) ;
#8650=EDGE_CURVE ( 'NONE', #10627, #10076, #6854, .T. ) ;
#8653=VECTOR ( 'NONE', #10665, 1000.000000000000114 ) ;
#8658=ORIENTED_EDGE ( 'NONE', *, *, #11285, .F. ) ;
#8668=VECTOR ( 'NONE', #23, 1000.000000000000000 ) ;
#8679=VECTOR ( 'NONE', #12654, 1000.000000000000000 ) ;
#8691=PLANE ( 'NONE',  #8907 ) ;
#8692=VERTEX_POINT ( 'NONE', #7610 ) ;
#8695=CARTESIAN_POINT ( 'NONE',  ( 50.00000000000000000, 40.00000000000000000, 0.000000000000000000 ) ) ;
#8702=DIRECTION ( 'NONE',  ( -1.000000000000000000, 0.000000000000000000, 0.000000000000000000 ) ) ;
#8721=CARTESIAN_POINT ( 'NONE',  ( -74.99999999999998579, -7.500000000000027534, 10.00000000000000000 ) ) ;
#8726=ADVANCED_FACE ( 'NONE', ( #1291, #11955 ), #1227, .T. ) ;
#8759=ORIENTED_EDGE ( 'NONE', *, *, #9205, .F. ) ;
#8766=DIRECTION ( 'NONE',  ( 1.000000000000000000, 0.000000000000000000, 0.000000000000000000 ) ) ;
#8778=CARTESIAN_POINT ( 'NONE',  ( -18.00000000000000355, -19.99999999999999289, -20.00000000000000000 ) ) ;
#8799=AXIS2_PLACEMENT_3D ( 'NONE', #8695, #1004, #2117 ) ;
#8806=CARTESIAN_POINT ( 'NONE',  ( 75.00000000000002842, -39.99999999999998579, 10.00000000000000000 ) ) ;
#8814=EDGE_CURVE ( 'NONE', #3281, #11826, #5949, .T. ) ;
#8835=CYLINDRICAL_SURFACE ( 'NONE', #9747, 12.50000000000000000 ) ;
#8847=DIRECTION ( 'NONE',  ( 0.000000000000000000, 1.000000000000000000, 0.000000000000000000 ) ) ;
#8856=CARTESIAN_POINT ( 'NONE',  ( -20.00000000000000000, -19.99999999999999289, -20.00000000000000000 ) ) ;
#8873=CARTESIAN_POINT ( 'NONE',  ( -7.499999999999998224, -20.00000000000000000, -10.00000000000000000 ) ) ;
#8906=CARTESIAN_POINT ( 'NONE',  ( 0.000000000000000000, 0.000000000000000000, -10.00000000000000000 ) ) ;
#8907=AXIS2_PLACEMENT_3D ( 'NONE', #9855, #3566, #8622 ) ;
#8915=ORIENTED_EDGE ( 'NONE', *, *, #1702, .F. ) ;
#8917=FACE_OUTER_BOUND ( 'NONE', #9217, .T. ) ;
#8933=ORIENTED_EDGE ( 'NONE', *, *, #5617, .T. ) ;
#8937=CYLINDRICAL_SURFACE ( 'NONE', #4782, 12.50000000000000000 ) ;
#8943=CARTESIAN_POINT ( 'NONE',  ( 30.00000000000000000, -7.499999999999971578, -10.00000000000000000 ) ) ;
#8946=EDGE_LOOP ( 'NONE', ( #7257, #2416, #3126, #10540 ) ) ;
#8967=CARTESIAN_POINT ( 'NONE',  ( -75.00000000000001421, -2.602085213965211904E-14, 0.000000000000000000 ) ) ;
#8969=DIRECTION ( 'NONE',  ( 0.000000000000000000, 1.000000000000000000, 0.000000000000000000 ) ) ;
#8976=VERTEX_POINT ( 'NONE', #6304 ) ;
#8979=LINE ( 'NONE', #12025, #9397 ) ;
#8981=ADVANCED_FACE ( 'NONE', ( #9460 ), #1993, .F. ) ;
#9003=CARTESIAN_POINT ( 'NONE',  ( -74.99999999999998579, -7.500000000000027534, -10.00000000000000000 ) ) ;
#9011=LINE ( 'NONE', #7979, #47 ) ;
#9014=VECTOR ( 'NONE', #7745, 1000.000000000000000 ) ;
#9016=EDGE_CURVE ( 'NONE', #11826, #1384, #13220, .T. ) ;
#9071=ADVANCED_FACE ( 'NONE', ( #12798 ), #2288, .F. ) ;
#9072=CARTESIAN_POINT ( 'NONE',  ( 30.00000000000000000, 1.040834085586084888E-14, 0.000000000000000000 ) ) ;
#9077=CARTESIAN_POINT ( 'NONE',  ( -74.99999999999998579, -2.602085213965210642E-14, 0.000000000000000000 ) ) ;
#9097=EDGE_CURVE ( 'NONE', #6230, #3838, #4195, .T. ) ;
#9100=ORIENTED_EDGE ( 'NONE', *, *, #1091, .T. ) ;
#9123=CARTESIAN_POINT ( 'NONE',  ( 18.00000000000000355, -20.00000000000000000, -20.00000000000000000 ) ) ;
#9134=ORIENTED_EDGE ( 'NONE', *, *, #4660, .F. ) ;
#9136=CARTESIAN_POINT ( 'NONE',  ( -74.99999999999997158, -7.499999999999971578, -10.00000000000000000 ) ) ;
#9156=CARTESIAN_POINT ( 'NONE',  ( -30.00000000000000000, -5.000000000000010658, 6.123233995736766282E-16 ) ) ;
#9163=AXIS2_PLACEMENT_3D ( 'NONE', #1633, #2610, #13116 ) ;
#9174=DIRECTION ( 'NONE',  ( -0.000000000000000000, -0.000000000000000000, -1.000000000000000000 ) ) ;
#9190=CARTESIAN_POINT ( 'NONE',  ( 50.00000000000000000, 40.00000000000000000, -4.000000000000003553 ) ) ;
#9205=EDGE_CURVE ( 'NONE', #11896, #1915, #6866, .T. ) ;
#9206=CARTESIAN_POINT ( 'NONE',  ( 2.449293598294706513E-15, -20.00000000000000000, -20.00000000000000000 ) ) ;
#9217=EDGE_LOOP ( 'NONE', ( #1845, #8188, #11482, #11145 ) ) ;
#9220=ORIENTED_EDGE ( 'NONE', *, *, #1877, .T. ) ;
#9228=DIRECTION ( 'NONE',  ( 1.000000000000000000, 0.000000000000000000, 0.000000000000000000 ) ) ;
#9236=ORIENTED_EDGE ( 'NONE', *, *, #9016, .F. ) ;
#9291=( NAMED_UNIT ( * ) PLANE_ANGLE_UNIT ( ) SI_UNIT ( $, .RADIAN. ) );
#9304=EDGE_CURVE ( 'NONE', #720, #8082, #1496, .T. ) ;
#9310=VECTOR ( 'NONE', #6892, 1000.000000000000000 ) ;
#9311=DIRECTION ( 'NONE',  ( -0.000000000000000000, -0.000000000000000000, -1.000000000000000000 ) ) ;
#9317=EDGE_CURVE ( 'NONE', #3838, #5822, #3797, .T. ) ;
#9325=ORIENTED_EDGE ( 'NONE', *, *, #2665, .F. ) ;
#9336=CARTESIAN_POINT ( 'NONE',  ( -74.99999999999997158, 40.00000000000001421, 10.00000000000000000 ) ) ;
#9340=VERTEX_POINT ( 'NONE', #11117 ) ;
#9343=ORIENTED_EDGE ( 'NONE', *, *, #5953, .T. ) ;
#9347=CARTESIAN_POINT ( 'NONE',  ( 2.449293598294706513E-15, -20.00000000000000000, -10.00000000000000000 ) ) ;
#9353=ADVANCED_FACE ( 'NONE', ( #6027 ), #11048, .F. ) ;
#9379=ORIENTED_EDGE ( 'NONE', *, *, #497, .T. ) ;
#9382=AXIS2_PLACEMENT_3D ( 'NONE', #5660, #9927, #640 ) ;
#9387=VECTOR ( 'NONE', #12393, 1000.000000000000000 ) ;
#9392=VECTOR ( 'NONE', #8354, 1000.000000000000000 ) ;
#9397=VECTOR ( 'NONE', #12158, 1000.000000000000000 ) ;
#9401=DIRECTION ( 'NONE',  ( -1.000000000000000000, 0.000000000000000000, 0.000000000000000000 ) ) ;
#9402=DIRECTION ( 'NONE',  ( 0.000000000000000000, -0.000000000000000000, 1.000000000000000000 ) ) ;
#9408=ORIENTED_EDGE ( 'NONE', *, *, #13588, .F. ) ;
#9409=EDGE_LOOP ( 'NONE', ( #423, #7569 ) ) ;
#9424=VERTEX_POINT ( 'NONE', #6101 ) ;
#9440=ORIENTED_EDGE ( 'NONE', *, *, #5741, .T. ) ;
#9455=ORIENTED_EDGE ( 'NONE', *, *, #1135, .T. ) ;
#9460=FACE_OUTER_BOUND ( 'NONE', #3684, .T. ) ;
#9473=DIRECTION ( 'NONE',  ( -0.000000000000000000, -0.000000000000000000, -1.000000000000000000 ) ) ;
#9494=AXIS2_PLACEMENT_3D ( 'NONE', #10277, #2152, #8528 ) ;
#9497=LINE ( 'NONE', #2093, #8668 ) ;
#9506=EDGE_CURVE ( 'NONE', #10021, #7078, #4867, .T. ) ;
#9519=EDGE_CURVE ( 'NONE', #686, #11745, #5327, .T. ) ;
#9523=VERTEX_POINT ( 'NONE', #3244 ) ;
#9526=FACE_BOUND ( 'NONE', #8204, .T. ) ;
#9544=CARTESIAN_POINT ( 'NONE',  ( -74.99999999999997158, 40.00000000000001421, -10.00000000000000000 ) ) ;
#9558=DIRECTION ( 'NONE',  ( 0.000000000000000000, 1.000000000000000000, 0.000000000000000000 ) ) ;
#9560=DIRECTION ( 'NONE',  ( -1.000000000000000000, 0.000000000000000000, 0.000000000000000000 ) ) ;
#9569=LINE ( 'NONE', #3275, #10291 ) ;
#9578=DIRECTION ( 'NONE',  ( -1.000000000000000000, 0.000000000000000000, 0.000000000000000000 ) ) ;
#9600=FACE_OUTER_BOUND ( 'NONE', #3419, .T. ) ;
#9605=VECTOR ( 'NONE', #2253, 1000.000000000000000 ) ;
#9610=EDGE_LOOP ( 'NONE', ( #4921, #11039, #3060, #9325 ) ) ;
#9622=VERTEX_POINT ( 'NONE', #8632 ) ;
#9626=DIRECTION ( 'NONE',  ( 0.000000000000000000, 0.000000000000000000, 1.000000000000000000 ) ) ;
#9628=LINE ( 'NONE', #10861, #3609 ) ;
#9639=ORIENTED_EDGE ( 'NONE', *, *, #10310, .F. ) ;
#9642=CYLINDRICAL_SURFACE ( 'NONE', #404, 5.000000000000000000 ) ;
#9643=EDGE_CURVE ( 'NONE', #5822, #13042, #218, .T. ) ;
#9656=EDGE_CURVE ( 'NONE', #3637, #2102, #6843, .T. ) ;
#9661=FACE_BOUND ( 'NONE', #12305, .T. ) ;
#9687=EDGE_LOOP ( 'NONE', ( #738, #13639, #13591, #5077 ) ) ;
#9707=DIRECTION ( 'NONE',  ( -1.000000000000000000, 0.000000000000000000, 0.000000000000000000 ) ) ;
#9709=PLANE ( 'NONE',  #4619 ) ;
#9716=VECTOR ( 'NONE', #4281, 1000.000000000000000 ) ;
#9728=EDGE_LOOP ( 'NONE', ( #6724, #11569, #5237, #6920 ) ) ;
#9735=ADVANCED_FACE ( 'NONE', ( #11806, #5731 ), #3581, .T. ) ;
#9747=AXIS2_PLACEMENT_3D ( 'NONE', #2739, #2595, #13032 ) ;
#9758=ORIENTED_EDGE ( 'NONE', *, *, #11753, .F. ) ;
#9761=DIRECTION ( 'NONE',  ( 0.000000000000000000, 0.000000000000000000, 1.000000000000000000 ) ) ;
#9779=CARTESIAN_POINT ( 'NONE',  ( 75.00000000000001421, -4.999999999999974243, 6.123233995736766282E-16 ) ) ;
#9794=EDGE_LOOP ( 'NONE', ( #9408, #5669, #8625, #11162, #7618, #4256, #2415, #1232 ) ) ;
#9801=DIRECTION ( 'NONE',  ( 1.000000000000000000, 3.469446951953615668E-16, -0.000000000000000000 ) ) ;
#9811=FACE_OUTER_BOUND ( 'NONE', #8147, .T. ) ;
#9826=ORIENTED_EDGE ( 'NONE', *, *, #11002, .T. ) ;
#9828=ORIENTED_EDGE ( 'NONE', *, *, #10636, .F. ) ;
#9841=ADVANCED_FACE ( 'NONE', ( #12281 ), #2743, .F. ) ;
#9842=CARTESIAN_POINT ( 'NONE',  ( -65.14999999999996305, 32.50000000000001421, -10.00000000000000178 ) ) ;
#9846=FACE_OUTER_BOUND ( 'NONE', #10869, .T. ) ;
#9855=CARTESIAN_POINT ( 'NONE',  ( -74.99999999999997158, 40.00000000000001421, 10.00000000000000000 ) ) ;
#9860=VECTOR ( 'NONE', #8592, 1000.000000000000000 ) ;
#9870=ORIENTED_EDGE ( 'NONE', *, *, #5617, .F. ) ;
#9872=CARTESIAN_POINT ( 'NONE',  ( 75.00000000000001421, 2.602085213965211904E-14, 0.000000000000000000 ) ) ;
#9890=EDGE_CURVE ( 'NONE', #1754, #8976, #9997, .T. ) ;
#9898=CIRCLE ( 'NONE', #830, 2.649999999999985700 ) ;
#9900=CYLINDRICAL_SURFACE ( 'NONE', #4932, 12.50000000000000000 ) ;
#9905=EDGE_LOOP ( 'NONE', ( #1714, #2946, #10120, #7553 ) ) ;
#9917=CARTESIAN_POINT ( 'NONE',  ( -29.99999999999999645, -40.00000000000000000, 10.00000000000000000 ) ) ;
#9925=AXIS2_PLACEMENT_3D ( 'NONE', #450, #2328, #10765 ) ;
#9927=DIRECTION ( 'NONE',  ( 0.000000000000000000, 0.000000000000000000, 1.000000000000000000 ) ) ;
#9944=VECTOR ( 'NONE', #5339, 1000.000000000000000 ) ;
#9945=CARTESIAN_POINT ( 'NONE',  ( -65.14999999999996305, 32.50000000000001421, 15.00000000000000000 ) ) ;
#9958=DIRECTION ( 'NONE',  ( -0.000000000000000000, -0.000000000000000000, -1.000000000000000000 ) ) ;
#9962=DIRECTION ( 'NONE',  ( 0.000000000000000000, 0.000000000000000000, -1.000000000000000000 ) ) ;
#9985=EDGE_LOOP ( 'NONE', ( #376, #8759 ) ) ;
#9986=EDGE_CURVE ( 'NONE', #2102, #3637, #5095, .T. ) ;
#9987=DIRECTION ( 'NONE',  ( 1.000000000000000000, 0.000000000000000000, 0.000000000000000000 ) ) ;
#9997=LINE ( 'NONE', #515, #8407 ) ;
#10021=VERTEX_POINT ( 'NONE', #11452 ) ;
#10023=CARTESIAN_POINT ( 'NONE',  ( 30.00000000000000355, 40.00000000000000000, 10.00000000000000000 ) ) ;
#10024=SHAPE_REPRESENTATION_RELATIONSHIP ( 'NONE' , 'NONE' ,  #10956, #5696 ) ;
#10076=VERTEX_POINT ( 'NONE', #10749 ) ;
#10120=ORIENTED_EDGE ( 'NONE', *, *, #7819, .T. ) ;
#10141=ADVANCED_FACE ( 'NONE', ( #4306 ), #11425, .T. ) ;
#10159=MANIFOLD_SOLID_BREP ( 'AdvancedHole2', #3608 ) ;
#10173=DIRECTION ( 'NONE',  ( -1.000000000000000000, -3.469446951953615175E-16, -0.000000000000000000 ) ) ;
#10200=VERTEX_POINT ( 'NONE', #12599 ) ;
#10228=ORIENTED_EDGE ( 'NONE', *, *, #13637, .F. ) ;
#10248=ORIENTED_EDGE ( 'NONE', *, *, #1952, .T. ) ;
#10258=AXIS2_PLACEMENT_3D ( 'NONE', #1778, #944, #9401 ) ;
#10277=CARTESIAN_POINT ( 'NONE',  ( -20.00000000000000000, -19.99999999999999289, -12.00000000000000000 ) ) ;
#10287=ORIENTED_EDGE ( 'NONE', *, *, #132, .F. ) ;
#10291=VECTOR ( 'NONE', #7635, 1000.000000000000000 ) ;
#10302=DIRECTION ( 'NONE',  ( -0.000000000000000000, -0.000000000000000000, 1.000000000000000000 ) ) ;
#10310=EDGE_CURVE ( 'NONE', #12157, #3807, #7624, .T. ) ;
#10328=LINE ( 'NONE', #699, #10432 ) ;
#10336=ORIENTED_EDGE ( 'NONE', *, *, #9656, .T. ) ;
#10339=VECTOR ( 'NONE', #1488, 1000.000000000000114 ) ;
#10351=ORIENTED_EDGE ( 'NONE', *, *, #8566, .T. ) ;
#10371=ORIENTED_EDGE ( 'NONE', *, *, #2536, .T. ) ;
#10398=AXIS2_PLACEMENT_3D ( 'NONE', #6795, #6663, #9962 ) ;
#10409=CARTESIAN_POINT ( 'NONE',  ( -20.00000000000000000, -19.99999999999999289, -10.79827876554711530 ) ) ;
#10410=DIRECTION ( 'NONE',  ( 0.000000000000000000, 0.000000000000000000, -1.000000000000000000 ) ) ;
#10427=ORIENTED_EDGE ( 'NONE', *, *, #1328, .T. ) ;
#10428=EDGE_CURVE ( 'NONE', #9622, #10987, #12173, .T. ) ;
#10432=VECTOR ( 'NONE', #3899, 1000.000000000000000 ) ;
#10443=AXIS2_PLACEMENT_3D ( 'NONE', #7623, #11827, #4574 ) ;
#10471=VECTOR ( 'NONE', #12601, 1000.000000000000000 ) ;
#10485=LINE ( 'NONE', #11534, #9392 ) ;
#10489=VERTEX_POINT ( 'NONE', #9136 ) ;
#10492=ORIENTED_EDGE ( 'NONE', *, *, #9317, .F. ) ;
#10498=DIRECTION ( 'NONE',  ( -1.000000000000000000, 0.000000000000000000, 0.000000000000000000 ) ) ;
#10500=EDGE_CURVE ( 'NONE', #7846, #10200, #6807, .T. ) ;
#10506=VERTEX_POINT ( 'NONE', #10023 ) ;
#10510=EDGE_CURVE ( 'NONE', #11165, #2102, #4851, .T. ) ;
#10512=CARTESIAN_POINT ( 'NONE',  ( 22.00000000000000000, -20.00000000000000000, -20.00000000000000000 ) ) ;
#10522=CIRCLE ( 'NONE', #3456, 12.50000000000000000 ) ;
#10526=DIRECTION ( 'NONE',  ( 1.000000000000000000, 3.469446951953615175E-16, 0.000000000000000000 ) ) ;
#10527=CARTESIAN_POINT ( 'NONE',  ( 30.00000000000000000, -40.00000000000000000, 12.50000000000000000 ) ) ;
#10540=ORIENTED_EDGE ( 'NONE', *, *, #4660, .T. ) ;
#10543=DIRECTION ( 'NONE',  ( -0.000000000000000000, -0.000000000000000000, -1.000000000000000000 ) ) ;
#10544=FACE_BOUND ( 'NONE', #941, .T. ) ;
#10554=EDGE_CURVE ( 'NONE', #5028, #8692, #1559, .T. ) ;
#10568=DIRECTION ( 'NONE',  ( -0.000000000000000000, 1.000000000000000000, -0.000000000000000000 ) ) ;
#10575=DIRECTION ( 'NONE',  ( 1.000000000000000000, 0.000000000000000000, 0.000000000000000000 ) ) ;
#10576=CONICAL_SURFACE ( 'NONE', #3514, 4.000000000000003553, 1.029744260000001077 ) ;
#10588=EDGE_CURVE ( 'NONE', #7078, #9424, #11182, .T. ) ;
#10590=ADVANCED_FACE ( 'NONE', ( #8917 ), #12973, .F. ) ;
#10625=ORIENTED_EDGE ( 'NONE', *, *, #13588, .T. ) ;
#10627=VERTEX_POINT ( 'NONE', #581 ) ;
#10631=DIRECTION ( 'NONE',  ( 0.000000000000000000, 0.000000000000000000, -1.000000000000000000 ) ) ;
#10636=EDGE_CURVE ( 'NONE', #13379, #4847, #597, .T. ) ;
#10647=DIRECTION ( 'NONE',  ( 1.000000000000000000, 0.000000000000000000, 0.000000000000000000 ) ) ;
#10654=LINE ( 'NONE', #5542, #7794 ) ;
#10665=DIRECTION ( 'NONE',  ( -0.8571673013836855759, 0.000000000000000000, -0.5150380737757258576 ) ) ;
#10667=AXIS2_PLACEMENT_3D ( 'NONE', #8856, #12166, #7890 ) ;
#10681=FACE_OUTER_BOUND ( 'NONE', #3993, .T. ) ;
#10693=CARTESIAN_POINT ( 'NONE',  ( 30.00000000000000000, 5.000000000000010658, 0.000000000000000000 ) ) ;
#10695=ORIENTED_EDGE ( 'NONE', *, *, #11603, .T. ) ;
#10702=CYLINDRICAL_SURFACE ( 'NONE', #3195, 5.000000000000000000 ) ;
#10711=ORIENTED_EDGE ( 'NONE', *, *, #7251, .F. ) ;
#10743=EDGE_CURVE ( 'NONE', #4149, #720, #9898, .T. ) ;
#10744=PRODUCT_DEFINITION_SHAPE ( 'NONE', 'NONE',  #4727 ) ;
#10749=CARTESIAN_POINT ( 'NONE',  ( 50.00000000000000000, 40.00000000000000000, -4.000000000000003553 ) ) ;
#10760=DIRECTION ( 'NONE',  ( 1.000000000000000000, 0.000000000000000000, 0.000000000000000000 ) ) ;
#10765=DIRECTION ( 'NONE',  ( -1.000000000000000000, 0.000000000000000000, -0.000000000000000000 ) ) ;
#10773=AXIS2_PLACEMENT_3D ( 'NONE', #3169, #11661, #5392 ) ;
#10801=AXIS2_PLACEMENT_3D ( 'NONE', #4006, #11187, #1637 ) ;
#10802=CARTESIAN_POINT ( 'NONE',  ( 20.00000000000000000, -20.00000000000000000, -12.00000000000000000 ) ) ;
#10805=AXIS2_PLACEMENT_3D ( 'NONE', #13204, #5772, #5838 ) ;
#10812=CARTESIAN_POINT ( 'NONE',  ( -74.99999999999997158, -7.500000000000027534, 10.00000000000000000 ) ) ;
#10834=EDGE_CURVE ( 'NONE', #9424, #5565, #3238, .T. ) ;
#10861=CARTESIAN_POINT ( 'NONE',  ( 75.00000000000001421, -7.499999999999971578, -20.00000000000000000 ) ) ;
#10862=AXIS2_PLACEMENT_3D ( 'NONE', #251, #9473, #6254 ) ;
#10869=EDGE_LOOP ( 'NONE', ( #6955, #4556, #1945, #3699 ) ) ;
#10900=EDGE_CURVE ( 'NONE', #10076, #10627, #11447, .T. ) ;
#10905=ADVANCED_FACE ( 'NONE', ( #5459, #9526, #9661, #7659 ), #7457, .T. ) ;
#10926=LINE ( 'NONE', #12790, #939 ) ;
#10929=( NAMED_UNIT ( * ) PLANE_ANGLE_UNIT ( ) SI_UNIT ( $, .RADIAN. ) );
#10931=CARTESIAN_POINT ( 'NONE',  ( -30.00000000000000000, -1.040834085586084257E-14, 0.000000000000000000 ) ) ;
#10956=SHAPE_REPRESENTATION ( 'Mounting block', ( #430 ), #11706 ) ;
#10962=CARTESIAN_POINT ( 'NONE',  ( 75.00000000000001421, -7.499999999999971578, -20.00000000000000000 ) ) ;
#10987=VERTEX_POINT ( 'NONE', #11096 ) ;
#10990=DIRECTION ( 'NONE',  ( 0.000000000000000000, 0.000000000000000000, 1.000000000000000000 ) ) ;
#10999=EDGE_CURVE ( 'NONE', #8692, #1384, #5863, .T. ) ;
#11002=EDGE_CURVE ( 'NONE', #3041, #8508, #11220, .T. ) ;
#11004=CYLINDRICAL_SURFACE ( 'NONE', #10805, 2.649999999999985700 ) ;
#11039=ORIENTED_EDGE ( 'NONE', *, *, #2899, .T. ) ;
#11048=CYLINDRICAL_SURFACE ( 'NONE', #10801, 1.999999999999998224 ) ;
#11057=ORIENTED_EDGE ( 'NONE', *, *, #2665, .T. ) ;
#11067=CYLINDRICAL_SURFACE ( 'NONE', #6480, 5.000000000000000000 ) ;
#11073=ADVANCED_FACE ( 'NONE', ( #7996 ), #7797, .F. ) ;
#11087=CARTESIAN_POINT ( 'NONE',  ( -74.99999999999998579, 7.499999999999975131, 10.00000000000000000 ) ) ;
#11096=CARTESIAN_POINT ( 'NONE',  ( 75.00000000000001421, -39.99999999999998579, -20.00000000000000000 ) ) ;
#11117=CARTESIAN_POINT ( 'NONE',  ( 50.00000000000000000, 15.00000000000000000, 4.000000000000003553 ) ) ;
#11131=CIRCLE ( 'NONE', #8506, 5.000000000000000000 ) ;
#11140=DIRECTION ( 'NONE',  ( 0.000000000000000000, 1.000000000000000000, 0.000000000000000000 ) ) ;
#11145=ORIENTED_EDGE ( 'NONE', *, *, #8814, .F. ) ;
#11157=CARTESIAN_POINT ( 'NONE',  ( 30.00000000000000000, -4.999999999999989342, 6.123233995736775157E-16 ) ) ;
#11162=ORIENTED_EDGE ( 'NONE', *, *, #1426, .F. ) ;
#11165=VERTEX_POINT ( 'NONE', #10409 ) ;
#11169=DIRECTION ( 'NONE',  ( -0.000000000000000000, -0.000000000000000000, 1.000000000000000000 ) ) ;
#11182=LINE ( 'NONE', #1701, #9014 ) ;
#11184=DIRECTION ( 'NONE',  ( 0.000000000000000000, 0.000000000000000000, -1.000000000000000000 ) ) ;
#11187=DIRECTION ( 'NONE',  ( -0.000000000000000000, -0.000000000000000000, -1.000000000000000000 ) ) ;
#11197=ORIENTED_EDGE ( 'NONE', *, *, #5699, .T. ) ;
#11212=ORIENTED_EDGE ( 'NONE', *, *, #9986, .F. ) ;
#11220=CIRCLE ( 'NONE', #12552, 12.50000000000000000 ) ;
#11242=CARTESIAN_POINT ( 'NONE',  ( 0.000000000000000000, 0.000000000000000000, 10.00000000000000000 ) ) ;
#11259=EDGE_CURVE ( 'NONE', #8692, #3281, #12121, .T. ) ;
#11261=ADVANCED_FACE ( 'NONE', ( #1120, #32 ), #9709, .F. ) ;
#11266=DIRECTION ( 'NONE',  ( 1.000000000000000000, -9.251858538542972814E-17, 0.000000000000000000 ) ) ;
#11270=VERTEX_POINT ( 'NONE', #12808 ) ;
#11277=DIRECTION ( 'NONE',  ( 0.000000000000000000, 1.000000000000000000, 0.000000000000000000 ) ) ;
#11283=ORIENTED_EDGE ( 'NONE', *, *, #12763, .F. ) ;
#11285=EDGE_CURVE ( 'NONE', #10489, #11319, #2179, .T. ) ;
#11288=ORIENTED_EDGE ( 'NONE', *, *, #12963, .F. ) ;
#11289=CARTESIAN_POINT ( 'NONE',  ( 75.00000000000001421, 7.500000000000027534, 10.00000000000000000 ) ) ;
#11319=VERTEX_POINT ( 'NONE', #7379 ) ;
#11325=DIRECTION ( 'NONE',  ( 1.000000000000000000, 0.000000000000000000, 0.000000000000000000 ) ) ;
#11344=CARTESIAN_POINT ( 'NONE',  ( 2.449293598294706513E-15, -20.00000000000000000, -10.00000000000000000 ) ) ;
#11354=ORIENTED_EDGE ( 'NONE', *, *, #13093, .T. ) ;
#11368=CIRCLE ( 'NONE', #7609, 5.000000000000000000 ) ;
#11377=ADVANCED_FACE ( 'NONE', ( #10681 ), #9642, .F. ) ;
#11382=PLANE ( 'NONE',  #7822 ) ;
#11396=CARTESIAN_POINT ( 'NONE',  ( 20.00000000000000000, -20.00000000000000000, -20.00000000000000000 ) ) ;
#11404=DIRECTION ( 'NONE',  ( -9.251858538542972814E-17, -1.000000000000000000, 0.000000000000000000 ) ) ;
#11414=DIRECTION ( 'NONE',  ( 0.000000000000000000, 1.000000000000000000, 0.000000000000000000 ) ) ;
#11425=CYLINDRICAL_SURFACE ( 'NONE', #3703, 12.50000000000000000 ) ;
#11434=( GEOMETRIC_REPRESENTATION_CONTEXT ( 3 ) GLOBAL_UNCERTAINTY_ASSIGNED_CONTEXT ( ( #6495 ) ) GLOBAL_UNIT_ASSIGNED_CONTEXT ( ( #3267, #9291, #4035 ) ) REPRESENTATION_CONTEXT ( 'NONE', 'WORKASPACE' ) );
#11447=CIRCLE ( 'NONE', #8799, 4.000000000000003553 ) ;
#11448=CARTESIAN_POINT ( 'NONE',  ( 0.000000000000000000, 0.000000000000000000, 10.00000000000000000 ) ) ;
#11449=CARTESIAN_POINT ( 'NONE',  ( -74.99999999999997158, -39.99999999999998579, 10.00000000000000000 ) ) ;
#11452=CARTESIAN_POINT ( 'NONE',  ( 75.00000000000001421, -7.499999999999971578, -10.00000000000000000 ) ) ;
#11462=CARTESIAN_POINT ( 'NONE',  ( -62.49999999999997158, 32.50000000000001421, -10.00000000000000178 ) ) ;
#11482=ORIENTED_EDGE ( 'NONE', *, *, #12275, .T. ) ;
#11486=DIRECTION ( 'NONE',  ( 0.000000000000000000, 0.000000000000000000, 1.000000000000000000 ) ) ;
#11511=AXIS2_PLACEMENT_3D ( 'NONE', #11771, #6532, #3136 ) ;
#11534=CARTESIAN_POINT ( 'NONE',  ( -74.99999999999997158, -39.99999999999998579, 10.00000000000000000 ) ) ;
#11539=ORIENTED_EDGE ( 'NONE', *, *, #10428, .T. ) ;
#11569=ORIENTED_EDGE ( 'NONE', *, *, #1702, .T. ) ;
#11573=DIRECTION ( 'NONE',  ( -0.000000000000000000, -1.000000000000000000, -0.000000000000000000 ) ) ;
#11603=EDGE_CURVE ( 'NONE', #6246, #2249, #13199, .T. ) ;
#11607=PLANE ( 'NONE',  #8068 ) ;
#11619=DIRECTION ( 'NONE',  ( 0.000000000000000000, 1.000000000000000000, 0.000000000000000000 ) ) ;
#11635=DIRECTION ( 'NONE',  ( -0.000000000000000000, 1.000000000000000000, -0.000000000000000000 ) ) ;
#11648=DIRECTION ( 'NONE',  ( 1.000000000000000000, 3.469446951953615175E-16, 0.000000000000000000 ) ) ;
#11661=DIRECTION ( 'NONE',  ( -0.000000000000000000, 0.000000000000000000, -1.000000000000000000 ) ) ;
#11669=ADVANCED_FACE ( 'NONE', ( #3942 ), #6317, .F. ) ;
#11671=AXIS2_PLACEMENT_3D ( 'NONE', #4332, #7516, #5383 ) ;
#11675=ORIENTED_EDGE ( 'NONE', *, *, #9506, .T. ) ;
#11681=CARTESIAN_POINT ( 'NONE',  ( 30.00000000000000000, 7.500000000000005329, -10.00000000000000711 ) ) ;
#11691=VERTEX_POINT ( 'NONE', #6109 ) ;
#11692=CARTESIAN_POINT ( 'NONE',  ( -74.99999999999997158, 40.00000000000001421, 10.00000000000000000 ) ) ;
#11706=( GEOMETRIC_REPRESENTATION_CONTEXT ( 3 ) GLOBAL_UNCERTAINTY_ASSIGNED_CONTEXT ( ( #6622 ) ) GLOBAL_UNIT_ASSIGNED_CONTEXT ( ( #2494, #10929, #7831 ) ) REPRESENTATION_CONTEXT ( 'NONE', 'WORKASPACE' ) );
#11714=CARTESIAN_POINT ( 'NONE',  ( 0.000000000000000000, 0.000000000000000000, 10.00000000000000000 ) ) ;
#11745=VERTEX_POINT ( 'NONE', #7134 ) ;
#11749=CARTESIAN_POINT ( 'NONE',  ( 2.449293598294706513E-15, -20.00000000000000000, -20.00000000000000000 ) ) ;
#11753=EDGE_CURVE ( 'NONE', #5220, #7288, #7283, .T. ) ;
#11765=DIRECTION ( 'NONE',  ( -0.000000000000000000, 1.000000000000000000, -0.000000000000000000 ) ) ;
#11771=CARTESIAN_POINT ( 'NONE',  ( 50.00000000000000000, 40.00000000000000000, 0.000000000000000000 ) ) ;
#11793=LINE ( 'NONE', #2316, #1156 ) ;
#11806=FACE_BOUND ( 'NONE', #7130, .T. ) ;
#11809=AXIS2_PLACEMENT_3D ( 'NONE', #13246, #13314, #11184 ) ;
#11817=EDGE_CURVE ( 'NONE', #13042, #5822, #2084, .T. ) ;
#11820=DIRECTION ( 'NONE',  ( -0.000000000000000000, 1.000000000000000000, -0.000000000000000000 ) ) ;
#11826=VERTEX_POINT ( 'NONE', #2474 ) ;
#11827=DIRECTION ( 'NONE',  ( 0.000000000000000000, 0.000000000000000000, -1.000000000000000000 ) ) ;
#11828=CARTESIAN_POINT ( 'NONE',  ( -29.99999999999999645, -39.99999999999998579, -12.49999999999999822 ) ) ;
#11829=FILL_AREA_STYLE_COLOUR ( '', #3108 ) ;
#11839=AXIS2_PLACEMENT_3D ( 'NONE', #9072, #3814, #12245 ) ;
#11853=EDGE_CURVE ( 'NONE', #8098, #3416, #11131, .T. ) ;
#11864=CARTESIAN_POINT ( 'NONE',  ( -74.99999999999997158, 40.00000000000001421, -10.00000000000000000 ) ) ;
#11865=DIRECTION ( 'NONE',  ( 0.000000000000000000, 0.000000000000000000, -1.000000000000000000 ) ) ;
#11879=VERTEX_POINT ( 'NONE', #12775 ) ;
#11881=AXIS2_PLACEMENT_3D ( 'NONE', #9872, #391, #8847 ) ;
#11882=ADVANCED_FACE ( 'NONE', ( #9811 ), #6512, .F. ) ;
#11895=EDGE_LOOP ( 'NONE', ( #5132, #9455, #669, #10695 ) ) ;
#11896=VERTEX_POINT ( 'NONE', #8778 ) ;
#11901=DIRECTION ( 'NONE',  ( 1.000000000000000000, -0.000000000000000000, -0.000000000000000000 ) ) ;
#11909=AXIS2_PLACEMENT_3D ( 'NONE', #13596, #8432, #9402 ) ;
#11955=FACE_OUTER_BOUND ( 'NONE', #7941, .T. ) ;
#11971=ORIENTED_EDGE ( 'NONE', *, *, #3344, .F. ) ;
#11989=AXIS2_PLACEMENT_3D ( 'NONE', #1924, #11404, #11266 ) ;
#12004=ORIENTED_EDGE ( 'NONE', *, *, #5437, .T. ) ;
#12005=ORIENTED_EDGE ( 'NONE', *, *, #12159, .F. ) ;
#12006=CARTESIAN_POINT ( 'NONE',  ( -20.00000000000000000, -19.99999999999999289, -20.00000000000000000 ) ) ;
#12022=ORIENTED_EDGE ( 'NONE', *, *, #216, .T. ) ;
#12025=CARTESIAN_POINT ( 'NONE',  ( -74.99999999999998579, 7.499999999999975131, 10.00000000000000000 ) ) ;
#12041=ORIENTED_EDGE ( 'NONE', *, *, #6895, .F. ) ;
#12055=FACE_OUTER_BOUND ( 'NONE', #9687, .T. ) ;
#12062=ADVANCED_FACE ( 'NONE', ( #4631, #7946 ), #6908, .F. ) ;
#12064=LINE ( 'NONE', #8059, #2335 ) ;
#12070=EDGE_CURVE ( 'NONE', #6246, #2319, #8979, .T. ) ;
#12104=AXIS2_PLACEMENT_3D ( 'NONE', #13133, #3675, #7897 ) ;
#12107=SURFACE_STYLE_FILL_AREA ( #7898 ) ;
#12121=CIRCLE ( 'NONE', #5730, 1.999999999999998224 ) ;
#12142=CARTESIAN_POINT ( 'NONE',  ( -74.99999999999997158, -39.99999999999998579, 10.00000000000000000 ) ) ;
#12156=DIRECTION ( 'NONE',  ( -1.000000000000000000, 0.000000000000000000, 0.000000000000000000 ) ) ;
#12157=VERTEX_POINT ( 'NONE', #583 ) ;
#12158=DIRECTION ( 'NONE',  ( 1.000000000000000000, 3.469446951953615175E-16, 0.000000000000000000 ) ) ;
#12159=EDGE_CURVE ( 'NONE', #3838, #6230, #4304, .T. ) ;
#12163=DIRECTION ( 'NONE',  ( 1.000000000000000000, 3.469446951953615668E-16, -0.000000000000000000 ) ) ;
#12166=DIRECTION ( 'NONE',  ( -0.000000000000000000, -0.000000000000000000, -1.000000000000000000 ) ) ;
#12173=LINE ( 'NONE', #5758, #1484 ) ;
#12205=ORIENTED_EDGE ( 'NONE', *, *, #9016, .T. ) ;
#12206=DIRECTION ( 'NONE',  ( -1.000000000000000000, 0.000000000000000000, 0.000000000000000000 ) ) ;
#12210=FACE_OUTER_BOUND ( 'NONE', #4607, .T. ) ;
#12245=DIRECTION ( 'NONE',  ( 0.000000000000000000, 0.000000000000000000, 1.000000000000000000 ) ) ;
#12275=EDGE_CURVE ( 'NONE', #1384, #11826, #4748, .T. ) ;
#12281=FACE_OUTER_BOUND ( 'NONE', #8946, .T. ) ;
#12299=DIRECTION ( 'NONE',  ( 1.000000000000000000, -0.000000000000000000, -0.000000000000000000 ) ) ;
#12303=ORIENTED_EDGE ( 'NONE', *, *, #2899, .F. ) ;
#12305=EDGE_LOOP ( 'NONE', ( #6691, #10248 ) ) ;
#12338=ORIENTED_EDGE ( 'NONE', *, *, #4754, .T. ) ;
#12349=DIRECTION ( 'NONE',  ( 0.000000000000000000, 0.000000000000000000, -1.000000000000000000 ) ) ;
#12380=FACE_OUTER_BOUND ( 'NONE', #11895, .T. ) ;
#12385=ADVANCED_FACE ( 'NONE', ( #183 ), #11607, .F. ) ;
#12393=DIRECTION ( 'NONE',  ( 1.000000000000000000, 3.469446951953615668E-16, -0.000000000000000000 ) ) ;
#12395=AXIS2_PLACEMENT_3D ( 'NONE', #366, #1461, #6742 ) ;
#12405=VECTOR ( 'NONE', #3945, 1000.000000000000000 ) ;
#12406=CARTESIAN_POINT ( 'NONE',  ( 50.00000000000000000, 40.00000000000000000, 4.000000000000003553 ) ) ;
#12426=ORIENTED_EDGE ( 'NONE', *, *, #7880, .T. ) ;
#12430=CARTESIAN_POINT ( 'NONE',  ( 20.00000000000000000, -20.00000000000000000, -20.00000000000000000 ) ) ;
#12434=PLANE ( 'NONE',  #11989 ) ;
#12436=ORIENTED_EDGE ( 'NONE', *, *, #1949, .F. ) ;
#12458=ORIENTED_EDGE ( 'NONE', *, *, #1426, .T. ) ;
#12459=VECTOR ( 'NONE', #298, 1000.000000000000000 ) ;
#12510=ORIENTED_EDGE ( 'NONE', *, *, #13451, .T. ) ;
#12512=CARTESIAN_POINT ( 'NONE',  ( -74.99999999999998579, -2.602085213965210642E-14, 0.000000000000000000 ) ) ;
#12516=CARTESIAN_POINT ( 'NONE',  ( 30.00000000000000355, 0.000000000000000000, -10.00000000000000000 ) ) ;
#12540=DIRECTION ( 'NONE',  ( -0.000000000000000000, -0.000000000000000000, 1.000000000000000000 ) ) ;
#12552=AXIS2_PLACEMENT_3D ( 'NONE', #12956, #9987, #3641 ) ;
#12559=DIRECTION ( 'NONE',  ( 0.000000000000000000, -1.000000000000000000, 0.000000000000000000 ) ) ;
#12564=ORIENTED_EDGE ( 'NONE', *, *, #2714, .F. ) ;
#12575=DIRECTION ( 'NONE',  ( 1.000000000000000000, -0.000000000000000000, -0.000000000000000000 ) ) ;
#12599=CARTESIAN_POINT ( 'NONE',  ( -30.00000000000000000, 4.999999999999989342, 0.000000000000000000 ) ) ;
#12601=DIRECTION ( 'NONE',  ( -0.000000000000000000, -0.000000000000000000, 1.000000000000000000 ) ) ;
#12612=DIRECTION ( 'NONE',  ( -1.000000000000000000, 0.000000000000000000, 0.000000000000000000 ) ) ;
#12613=ORIENTED_EDGE ( 'NONE', *, *, #1226, .F. ) ;
#12615=ORIENTED_EDGE ( 'NONE', *, *, #6676, .T. ) ;
#12646=ORIENTED_EDGE ( 'NONE', *, *, #4640, .T. ) ;
#12654=DIRECTION ( 'NONE',  ( -1.000000000000000000, -3.469446951953615175E-16, -0.000000000000000000 ) ) ;
#12662=LINE ( 'NONE', #7364, #4965 ) ;
#12691=DIRECTION ( 'NONE',  ( -0.000000000000000000, -0.000000000000000000, 1.000000000000000000 ) ) ;
#12704=DIRECTION ( 'NONE',  ( 0.000000000000000000, 1.000000000000000000, 0.000000000000000000 ) ) ;
#12706=ADVANCED_FACE ( 'NONE', ( #2948 ), #11382, .F. ) ;
#12721=PRODUCT ( 'Mounting block', 'Mounting block', '', ( #6129 ) ) ;
#12741=PLANE ( 'NONE',  #1846 ) ;
#12757=DIRECTION ( 'NONE',  ( -1.000000000000000000, 9.251858538542972814E-17, -0.000000000000000000 ) ) ;
#12762=CARTESIAN_POINT ( 'NONE',  ( -74.99999999999997158, -39.99999999999998579, -10.00000000000000000 ) ) ;
#12763=EDGE_CURVE ( 'NONE', #9523, #9424, #4054, .T. ) ;
#12766=EDGE_CURVE ( 'NONE', #3637, #1915, #2040, .T. ) ;
#12775=CARTESIAN_POINT ( 'NONE',  ( -30.00000000000000000, -7.500000000000011546, 10.00000000000000000 ) ) ;
#12777=CIRCLE ( 'NONE', #13212, 1.999999999999998224 ) ;
#12786=ORIENTED_EDGE ( 'NONE', *, *, #1091, .F. ) ;
#12790=CARTESIAN_POINT ( 'NONE',  ( 50.00000000000000000, 15.00000000000000000, -4.000000000000003553 ) ) ;
#12798=FACE_OUTER_BOUND ( 'NONE', #5718, .T. ) ;
#12808=CARTESIAN_POINT ( 'NONE',  ( 30.00000000000000000, 7.500000000000011546, 10.00000000000000000 ) ) ;
#12824=ORIENTED_EDGE ( 'NONE', *, *, #10743, .F. ) ;
#12841=ORIENTED_EDGE ( 'NONE', *, *, #6676, .F. ) ;
#12857=FACE_OUTER_BOUND ( 'NONE', #9728, .T. ) ;
#12870=EDGE_LOOP ( 'NONE', ( #5825, #12041, #1486, #13313 ) ) ;
#12878=ADVANCED_FACE ( 'NONE', ( #10544, #236 ), #12741, .F. ) ;
#12886=DIRECTION ( 'NONE',  ( -0.000000000000000000, -1.000000000000000000, -0.000000000000000000 ) ) ;
#12897=CARTESIAN_POINT ( 'NONE',  ( -75.00000000000001421, -2.602085213965211904E-14, 0.000000000000000000 ) ) ;
#12909=ORIENTED_EDGE ( 'NONE', *, *, #12766, .F. ) ;
#12911=DIRECTION ( 'NONE',  ( -0.000000000000000000, 1.000000000000000000, -0.000000000000000000 ) ) ;
#12919=VERTEX_POINT ( 'NONE', #2370 ) ;
#12922=VERTEX_POINT ( 'NONE', #8414 ) ;
#12925=CARTESIAN_POINT ( 'NONE',  ( -65.14999999999996305, 32.50000000000001421, 10.00000000000000000 ) ) ;
#12931=VECTOR ( 'NONE', #24, 1000.000000000000000 ) ;
#12953=EDGE_LOOP ( 'NONE', ( #7844, #10625, #12564, #2959 ) ) ;
#12956=CARTESIAN_POINT ( 'NONE',  ( 30.00000000000000000, 1.040834085586084888E-14, 0.000000000000000000 ) ) ;
#12960=DIRECTION ( 'NONE',  ( -3.469446951953614682E-16, 1.000000000000000000, 0.000000000000000000 ) ) ;
#12963=EDGE_CURVE ( 'NONE', #720, #4149, #726, .T. ) ;
#12973=CYLINDRICAL_SURFACE ( 'NONE', #13641, 1.999999999999998224 ) ;
#12979=AXIS2_PLACEMENT_3D ( 'NONE', #8094, #12299, #2831 ) ;
#12987=AXIS2_PLACEMENT_3D ( 'NONE', #9206, #10302, #10575 ) ;
#13012=CARTESIAN_POINT ( 'NONE',  ( 75.00000000000001421, -7.499999999999971578, -10.00000000000000000 ) ) ;
#13023=FACE_OUTER_BOUND ( 'NONE', #6459, .T. ) ;
#13026=VERTEX_POINT ( 'NONE', #3421 ) ;
#13032=DIRECTION ( 'NONE',  ( 0.000000000000000000, 1.000000000000000000, 0.000000000000000000 ) ) ;
#13042=VERTEX_POINT ( 'NONE', #9779 ) ;
#13065=( NAMED_UNIT ( * ) SI_UNIT ( $, .STERADIAN. ) SOLID_ANGLE_UNIT ( ) );
#13066=DIRECTION ( 'NONE',  ( -0.000000000000000000, -0.000000000000000000, 1.000000000000000000 ) ) ;
#13091=EDGE_LOOP ( 'NONE', ( #12613, #5058, #12615, #5615 ) ) ;
#13093=EDGE_CURVE ( 'NONE', #10489, #12919, #7978, .T. ) ;
#13100=DIRECTION ( 'NONE',  ( -1.000000000000000000, 0.000000000000000000, 0.000000000000000000 ) ) ;
#13116=DIRECTION ( 'NONE',  ( 0.000000000000000000, 0.000000000000000000, -1.000000000000000000 ) ) ;
#13118=CIRCLE ( 'NONE', #312, 12.50000000000000000 ) ;
#13133=CARTESIAN_POINT ( 'NONE',  ( -30.00000000000000000, -1.040834085586084257E-14, 0.000000000000000000 ) ) ;
#13147=CARTESIAN_POINT ( 'NONE',  ( -74.99999999999997158, -39.99999999999998579, 10.00000000000000000 ) ) ;
#13165=EDGE_CURVE ( 'NONE', #1754, #9622, #3756, .T. ) ;
#13199=CIRCLE ( 'NONE', #13653, 12.50000000000000000 ) ;
#13204=CARTESIAN_POINT ( 'NONE',  ( -62.49999999999997158, 32.50000000000001421, 15.00000000000000000 ) ) ;
#13212=AXIS2_PLACEMENT_3D ( 'NONE', #10802, #6670, #9707 ) ;
#13220=CIRCLE ( 'NONE', #8605, 1.999999999999998224 ) ;
#13226=CARTESIAN_POINT ( 'NONE',  ( 22.00000000000000000, -20.00000000000000000, -20.00000000000000000 ) ) ;
#13246=CARTESIAN_POINT ( 'NONE',  ( 30.00000000000000000, 1.040834085586084888E-14, 0.000000000000000000 ) ) ;
#13313=ORIENTED_EDGE ( 'NONE', *, *, #6713, .F. ) ;
#13314=DIRECTION ( 'NONE',  ( -1.000000000000000000, 0.000000000000000000, -0.000000000000000000 ) ) ;
#13363=ORIENTED_EDGE ( 'NONE', *, *, #10428, .F. ) ;
#13379=VERTEX_POINT ( 'NONE', #11289 ) ;
#13381=DIRECTION ( 'NONE',  ( -1.000000000000000000, 0.000000000000000000, 0.000000000000000000 ) ) ;
#13397=DIRECTION ( 'NONE',  ( 0.000000000000000000, 1.000000000000000000, 0.000000000000000000 ) ) ;
#13401=DIRECTION ( 'NONE',  ( 0.000000000000000000, 1.000000000000000000, 0.000000000000000000 ) ) ;
#13416=LINE ( 'NONE', #3960, #9387 ) ;
#13451=EDGE_CURVE ( 'NONE', #3416, #7846, #13416, .T. ) ;
#13489=ADVANCED_FACE ( 'NONE', ( #13624, #8458 ), #82, .T. ) ;
#13527=EDGE_CURVE ( 'NONE', #11879, #3807, #12662, .T. ) ;
#13547=VECTOR ( 'NONE', #9311, 1000.000000000000000 ) ;
#13550=CONICAL_SURFACE ( 'NONE', #1624, 1.999999999999998224, 1.029744259999999745 ) ;
#13576=VERTEX_POINT ( 'NONE', #7428 ) ;
#13588=EDGE_CURVE ( 'NONE', #5565, #10506, #4171, .T. ) ;
#13591=ORIENTED_EDGE ( 'NONE', *, *, #134, .F. ) ;
#13593=ADVANCED_FACE ( 'NONE', ( #152 ), #4507, .F. ) ;
#13596=CARTESIAN_POINT ( 'NONE',  ( -74.99999999999997158, -39.99999999999998579, 10.00000000000000000 ) ) ;
#13602=VECTOR ( 'NONE', #11414, 1000.000000000000000 ) ;
#13611=LINE ( 'NONE', #5272, #8226 ) ;
#13624=FACE_OUTER_BOUND ( 'NONE', #9794, .T. ) ;
#13629=STYLED_ITEM('',(#13684),#10159);
#13635=FACE_OUTER_BOUND ( 'NONE', #7549, .T. ) ;
#13637=EDGE_CURVE ( 'NONE', #966, #686, #3268, .T. ) ;
#13638=LINE ( 'NONE', #12406, #2115 ) ;
#13639=ORIENTED_EDGE ( 'NONE', *, *, #9304, .T. ) ;
#13640=DIRECTION ( 'NONE',  ( -1.000000000000000000, -3.469446951953615175E-16, 0.000000000000000000 ) ) ;
#13641=AXIS2_PLACEMENT_3D ( 'NONE', #1631, #3520, #12156 ) ;
#13653=AXIS2_PLACEMENT_3D ( 'NONE', #12512, #8375, #13397 ) ;
#13678=COLOUR_RGB('Dark Blue',0.08,0.2,0.34);
#13679=FILL_AREA_STYLE_COLOUR('',#13678);
#13680=FILL_AREA_STYLE('',(#13679));
#13681=SURFACE_STYLE_FILL_AREA(#13680);
#13682=SURFACE_SIDE_STYLE('',(#13681));
#13683=SURFACE_STYLE_USAGE(.BOTH.,#13682);
#13684=PRESENTATION_STYLE_ASSIGNMENT((#13683));
ENDSEC;
END-ISO-10303-21;
